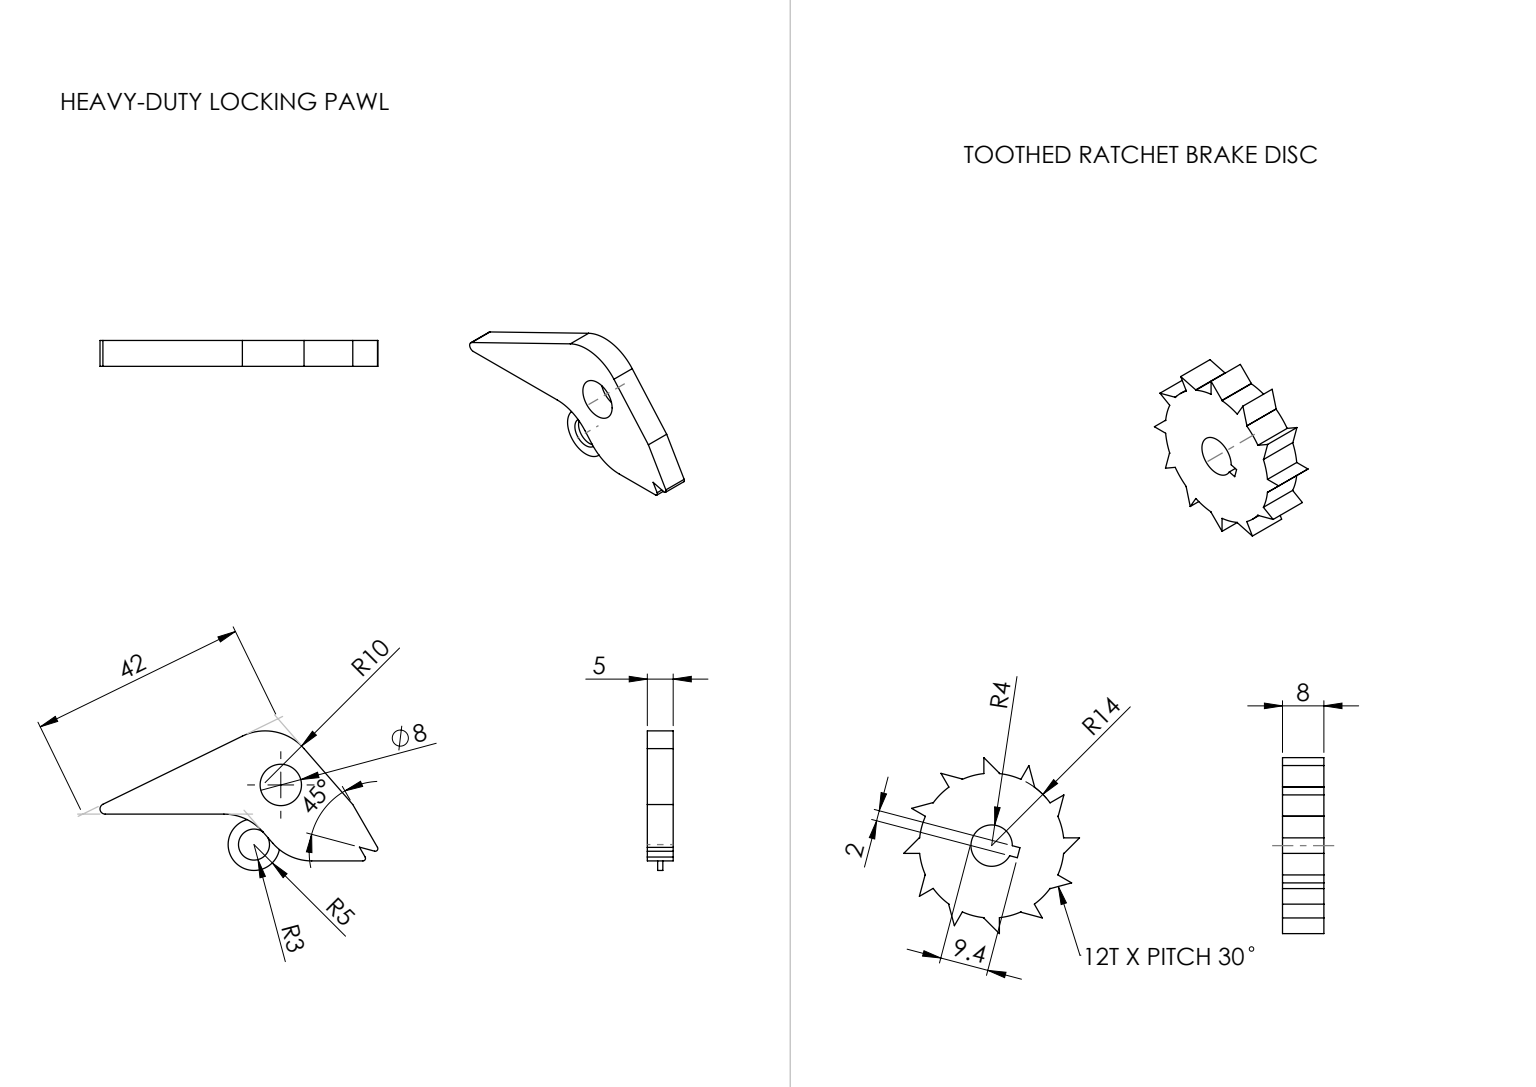
ISO-10303-21;
HEADER;
FILE_DESCRIPTION (('STEP AP214'),
    '1' );
FILE_NAME ('Toothed Ratchet Brake Disc.step',
    '2026-09-28T15:49:00',
    ( '' ),
    ( '' ),
    'SwSTEP 2.0',
    'SolidWorks 2026',
    '' );
FILE_SCHEMA (( 'AUTOMOTIVE_DESIGN' ));
ENDSEC;

DATA;
#67=DIRECTION ( 'NONE',  ( 1.226634733346697831E-16, 0.9659258262890664248, 0.2588190451025275673 ) ) ;
#91=SURFACE_STYLE_FILL_AREA ( #262 ) ;
#100=SURFACE_STYLE_FILL_AREA ( #24773 ) ;
#106=AXIS2_PLACEMENT_3D ( 'NONE', #28368, #3711, #14664 ) ;
#138=VECTOR ( 'NONE', #11051, 999.9999999999998863 ) ;
#168=DIRECTION ( 'NONE',  ( 0.000000000000000000, -2.423959199780483078E-15, 1.000000000000000000 ) ) ;
#214=CARTESIAN_POINT ( 'NONE',  ( -34.49999999999998579, -13.17619866229204284, 90.66066734786082293 ) ) ;
#223=VERTEX_POINT ( 'NONE', #1907 ) ;
#230=EDGE_CURVE ( 'NONE', #16800, #15848, #17909, .T. ) ;
#248=LINE ( 'NONE', #32677, #17648 ) ;
#262=FILL_AREA_STYLE ('',( #8710 ) ) ;
#273=CARTESIAN_POINT ( 'NONE',  ( -21.15833593587365513, -18.77980021920990694, 100.4724318643354053 ) ) ;
#283=CARTESIAN_POINT ( 'NONE',  ( -42.49999999999999289, -34.23950567274748380, 96.30456345124107997 ) ) ;
#289=VECTOR ( 'NONE', #25912, 1000.000000000000000 ) ;
#294=CARTESIAN_POINT ( 'NONE',  ( -42.49999999999999289, -25.98076211353322051, 84.99999999999992895 ) ) ;
#298=CARTESIAN_POINT ( 'NONE',  ( -34.49999999999998579, -28.81745899286249823, 74.41330312067046293 ) ) ;
#300=ADVANCED_FACE ( 'NONE', ( #12882 ), #23862, .F. ) ;
#305=CARTESIAN_POINT ( 'NONE',  ( -21.15833593587365513, -33.18172400785640264, 69.52756813566438154 ) ) ;
#336=ORIENTED_EDGE ( 'NONE', *, *, #17121, .F. ) ;
#370=AXIS2_PLACEMENT_3D ( 'NONE', #13032, #24546, #7606 ) ;
#374=DIRECTION ( 'NONE',  ( -1.226634733346697831E-16, -0.2588190451025116356, -0.9659258262890706437 ) ) ;
#376=EDGE_LOOP ( 'NONE', ( #21433, #15135, #23914, #10868 ) ) ;
#381=DIRECTION ( 'NONE',  ( 1.000000000000000000, 0.000000000000000000, 0.000000000000000000 ) ) ;
#391=ORIENTED_EDGE ( 'NONE', *, *, #34173, .T. ) ;
#484=CARTESIAN_POINT ( 'NONE',  ( -34.49999999999998579, -34.23950567274747669, 96.30456345124106576 ) ) ;
#490=ORIENTED_EDGE ( 'NONE', *, *, #31210, .T. ) ;
#532=VERTEX_POINT ( 'NONE', #20194 ) ;
#590=VECTOR ( 'NONE', #2265, 1000.000000000000000 ) ;
#612=SURFACE_SIDE_STYLE ('',( #91 ) ) ;
#625=DIRECTION ( 'NONE',  ( 0.000000000000000000, 1.000000000000000000, 0.000000000000000000 ) ) ;
#642=CARTESIAN_POINT ( 'NONE',  ( -21.15833593587365513, -14.60640646055094649, 76.70096189432339884 ) ) ;
#659=CARTESIAN_POINT ( 'NONE',  ( -34.49999999999998579, -25.98076211353320986, 84.99999999999994316 ) ) ;
#697=VECTOR ( 'NONE', #11975, 1000.000000000000114 ) ;
#709=VECTOR ( 'NONE', #30336, 1000.000000000000000 ) ;
#713=ORIENTED_EDGE ( 'NONE', *, *, #23446, .F. ) ;
#720=CARTESIAN_POINT ( 'NONE',  ( -42.49999999999999289, -12.06135120645816983, 86.49999999999994316 ) ) ;
#743=EDGE_CURVE ( 'NONE', #35591, #7199, #12479, .T. ) ;
#745=EDGE_CURVE ( 'NONE', #21122, #17030, #7068, .T. ) ;
#746=DIRECTION ( 'NONE',  ( 0.000000000000000000, -0.4999999999999958367, -0.8660254037844410391 ) ) ;
#747=VECTOR ( 'NONE', #16758, 1000.000000000000000 ) ;
#750=EDGE_LOOP ( 'NONE', ( #4388, #25058, #30347, #34872, #28090, #6286 ) ) ;
#767=CARTESIAN_POINT ( 'NONE',  ( -21.15833593587365513, -26.68172400785662290, 89.21410161513769310 ) ) ;
#789=PRESENTATION_STYLE_ASSIGNMENT (( #11768 ) ) ;
#793=VERTEX_POINT ( 'NONE', #28863 ) ;
#820=ORIENTED_EDGE ( 'NONE', *, *, #33243, .T. ) ;
#830=ORIENTED_EDGE ( 'NONE', *, *, #13493, .F. ) ;
#861=CARTESIAN_POINT ( 'NONE',  ( -34.49999999999998579, -25.98076211353322051, 84.99999999999992895 ) ) ;
#872=PRODUCT_DEFINITION_SHAPE ( 'NONE', 'NONE',  #912 ) ;
#874=AXIS2_PLACEMENT_3D ( 'NONE', #19196, #30544, #22421 ) ;
#882=CARTESIAN_POINT ( 'NONE',  ( -34.49999999999998579, -31.64142946139415713, 97.80456345124107997 ) ) ;
#884=ORIENTED_EDGE ( 'NONE', *, *, #5572, .F. ) ;
#912=PRODUCT_DEFINITION ( 'UNKNOWN', '', #34489, #31011 ) ;
#916=LINE ( 'NONE', #17108, #747 ) ;
#930=VECTOR ( 'NONE', #2407, 1000.000000000000114 ) ;
#952=DIRECTION ( 'NONE',  ( 0.000000000000000000, 0.8660254037844444808, -0.4999999999999898415 ) ) ;
#957=UNCERTAINTY_MEASURE_WITH_UNIT (LENGTH_MEASURE( 1.000000000000000082E-05 ), #30348, 'distance_accuracy_value', 'NONE');
#969=DIRECTION ( 'NONE',  ( -1.734723475976807094E-16, 0.8660254037844444808, -0.4999999999999898415 ) ) ;
#1011=CARTESIAN_POINT ( 'NONE',  ( -42.49999999999999289, -28.69486372867094559, 81.70096189432321410 ) ) ;
#1039=ORIENTED_EDGE ( 'NONE', *, *, #33488, .T. ) ;
#1041=CARTESIAN_POINT ( 'NONE',  ( -34.49999999999998579, -25.98076211353322051, 84.99999999999992895 ) ) ;
#1058=DIRECTION ( 'NONE',  ( 0.000000000000000000, -1.000000000000000000, 1.067522139062650474E-15 ) ) ;
#1064=EDGE_CURVE ( 'NONE', #1802, #27521, #4812, .T. ) ;
#1077=CARTESIAN_POINT ( 'NONE',  ( -34.49999999999998579, -25.98076211353322051, 84.99999999999992895 ) ) ;
#1084=FACE_OUTER_BOUND ( 'NONE', #26395, .T. ) ;
#1107=ORIENTED_EDGE ( 'NONE', *, *, #7172, .T. ) ;
#1108=LINE ( 'NONE', #12077, #15873 ) ;
#1118=ORIENTED_EDGE ( 'NONE', *, *, #2748, .F. ) ;
#1133=EDGE_CURVE ( 'NONE', #14117, #4018, #916, .T. ) ;
#1135=DIRECTION ( 'NONE',  ( -1.000000000000000000, -1.734723475976807094E-16, -0.000000000000000000 ) ) ;
#1160=ORIENTED_EDGE ( 'NONE', *, *, #5332, .F. ) ;
#1190=DIRECTION ( 'NONE',  ( -1.000000000000000000, -1.734723475976807094E-16, -0.000000000000000000 ) ) ;
#1231=VECTOR ( 'NONE', #22493, 1000.000000000000000 ) ;
#1252=ORIENTED_EDGE ( 'NONE', *, *, #745, .F. ) ;
#1254=EDGE_CURVE ( 'NONE', #9156, #35591, #5972, .T. ) ;
#1256=VERTEX_POINT ( 'NONE', #17999 ) ;
#1281=ORIENTED_EDGE ( 'NONE', *, *, #9466, .T. ) ;
#1292=CARTESIAN_POINT ( 'NONE',  ( -42.49999999999999289, -27.48076211353326670, 88.99999999999994316 ) ) ;
#1302=DIRECTION ( 'NONE',  ( -1.000000000000000000, 8.673617379884106963E-17, -1.502314598737155580E-16 ) ) ;
#1323=AXIS2_PLACEMENT_3D ( 'NONE', #31219, #31395, #28341 ) ;
#1325=CARTESIAN_POINT ( 'NONE',  ( -34.49999999999998579, -25.98076211353322051, 84.99999999999992895 ) ) ;
#1350=LINE ( 'NONE', #28720, #24089 ) ;
#1363=CARTESIAN_POINT ( 'NONE',  ( -42.49999999999999289, -28.31857036507959791, 80.03062855292519373 ) ) ;
#1377=ORIENTED_EDGE ( 'NONE', *, *, #12991, .T. ) ;
#1445=LINE ( 'NONE', #31682, #19350 ) ;
#1448=VECTOR ( 'NONE', #31600, 1000.000000000000000 ) ;
#1470=CARTESIAN_POINT ( 'NONE',  ( -42.49999999999999289, -39.98076211353324538, 86.49999999999991473 ) ) ;
#1481=VECTOR ( 'NONE', #20731, 1000.000000000000114 ) ;
#1493=PLANE ( 'NONE',  #24055 ) ;
#1540=PLANE ( 'NONE',  #18233 ) ;
#1549=LINE ( 'NONE', #34863, #34826 ) ;
#1578=CARTESIAN_POINT ( 'NONE',  ( -34.49999999999998579, -25.98076211353322051, 84.99999999999992895 ) ) ;
#1582=EDGE_CURVE ( 'NONE', #13818, #6950, #20310, .T. ) ;
#1596=ORIENTED_EDGE ( 'NONE', *, *, #33710, .T. ) ;
#1623=ORIENTED_EDGE ( 'NONE', *, *, #17089, .F. ) ;
#1665=EDGE_CURVE ( 'NONE', #29583, #1876, #28085, .T. ) ;
#1668=EDGE_LOOP ( 'NONE', ( #2169, #17743, #21622, #22182 ) ) ;
#1721=DIRECTION ( 'NONE',  ( -1.000000000000000000, -1.734723475976807094E-16, -0.000000000000000000 ) ) ;
#1722=ORIENTED_EDGE ( 'NONE', *, *, #30631, .F. ) ;
#1723=CARTESIAN_POINT ( 'NONE',  ( -34.49999999999998579, -29.98076211353321341, 84.99999999999994316 ) ) ;
#1745=EDGE_CURVE ( 'NONE', #7407, #24192, #5764, .T. ) ;
#1747=CIRCLE ( 'NONE', #6335, 14.00000000000000000 ) ;
#1771=ORIENTED_EDGE ( 'NONE', *, *, #20086, .T. ) ;
#1772=VECTOR ( 'NONE', #28510, 1000.000000000000000 ) ;
#1790=SHAPE_REPRESENTATION ( 'Toothed Ratchet Brake Disc', ( #21307 ), #24207 ) ;
#1796=EDGE_LOOP ( 'NONE', ( #2648, #490, #8320, #32587 ) ) ;
#1798=LINE ( 'NONE', #15450, #30635 ) ;
#1802=VERTEX_POINT ( 'NONE', #20830 ) ;
#1849=DIRECTION ( 'NONE',  ( -1.734723475976807094E-16, -1.000000000000000000, 1.067522139062650474E-15 ) ) ;
#1861=LINE ( 'NONE', #9769, #1481 ) ;
#1876=VERTEX_POINT ( 'NONE', #34375 ) ;
#1897=CARTESIAN_POINT ( 'NONE',  ( -21.15833593587365513, -17.68172400785659448, 96.37435565298210349 ) ) ;
#1907=CARTESIAN_POINT ( 'NONE',  ( -34.49999999999998579, -20.27980021920970799, 72.12564434701783966 ) ) ;
#1942=CARTESIAN_POINT ( 'NONE',  ( -34.49999999999998579, -25.98076211353322051, 84.99999999999992895 ) ) ;
#1944=LINE ( 'NONE', #4657, #30693 ) ;
#1993=DIRECTION ( 'NONE',  ( -1.734723475976806848E-16, -0.5000000000000032196, 0.8660254037844368202 ) ) ;
#2045=ADVANCED_FACE ( 'NONE', ( #10242 ), #21015, .F. ) ;
#2055=CARTESIAN_POINT ( 'NONE',  ( -21.15833593587365513, -41.45319397786874305, 92.20096189432315725 ) ) ;
#2065=AXIS2_PLACEMENT_3D ( 'NONE', #10185, #21155, #35049 ) ;
#2089=LINE ( 'NONE', #5145, #15629 ) ;
#2128=VECTOR ( 'NONE', #14487, 1000.000000000000114 ) ;
#2135=DIRECTION ( 'NONE',  ( 0.000000000000000000, 1.000000000000000000, 0.000000000000000000 ) ) ;
#2143=DIRECTION ( 'NONE',  ( -1.000000000000000000, 0.000000000000000000, 0.000000000000000000 ) ) ;
#2158=VERTEX_POINT ( 'NONE', #5888 ) ;
#2167=CIRCLE ( 'NONE', #11345, 4.000000000000003553 ) ;
#2169=ORIENTED_EDGE ( 'NONE', *, *, #33690, .T. ) ;
#2219=EDGE_CURVE ( 'NONE', #1802, #4018, #27520, .T. ) ;
#2233=EDGE_LOOP ( 'NONE', ( #14028, #3994, #27129, #18101 ) ) ;
#2265=DIRECTION ( 'NONE',  ( 0.000000000000000000, 0.8660254037844444808, -0.4999999999999898415 ) ) ;
#2267=EDGE_CURVE ( 'NONE', #21074, #13818, #12004, .T. ) ;
#2275=LINE ( 'NONE', #13243, #709 ) ;
#2302=EDGE_CURVE ( 'NONE', #19176, #17996, #9826, .T. ) ;
#2303=FACE_OUTER_BOUND ( 'NONE', #6582, .T. ) ;
#2316=DIRECTION ( 'NONE',  ( -1.000000000000000000, -8.673617379884000959E-17, -1.502314598737161250E-16 ) ) ;
#2346=AXIS2_PLACEMENT_3D ( 'NONE', #11575, #33536, #11404 ) ;
#2383=( GEOMETRIC_REPRESENTATION_CONTEXT ( 3 ) GLOBAL_UNCERTAINTY_ASSIGNED_CONTEXT ( ( #20016 ) ) GLOBAL_UNIT_ASSIGNED_CONTEXT ( ( #33391, #27658, #14121 ) ) REPRESENTATION_CONTEXT ( 'NONE', 'WORKASPACE' ) );
#2407=DIRECTION ( 'NONE',  ( 1.226634733346697831E-16, -0.9659258262890715319, 0.2588190451025083605 ) ) ;
#2456=VERTEX_POINT ( 'NONE', #10009 ) ;
#2462=EDGE_CURVE ( 'NONE', #20834, #17030, #15565, .T. ) ;
#2484=CARTESIAN_POINT ( 'NONE',  ( -21.15833593587365513, -27.48076211353304998, 70.99999999999988631 ) ) ;
#2498=VERTEX_POINT ( 'NONE', #32328 ) ;
#2517=DIRECTION ( 'NONE',  ( -1.000000000000000000, 0.000000000000000000, 0.000000000000000000 ) ) ;
#2520=EDGE_CURVE ( 'NONE', #32530, #7199, #35056, .T. ) ;
#2523=EDGE_CURVE ( 'NONE', #4350, #6950, #13086, .T. ) ;
#2530=CARTESIAN_POINT ( 'NONE',  ( -42.49999999999999289, -29.98076211353323828, 83.49999999999990052 ) ) ;
#2555=AXIS2_PLACEMENT_3D ( 'NONE', #6224, #11791, #31419 ) ;
#2578=VERTEX_POINT ( 'NONE', #3343 ) ;
#2602=CIRCLE ( 'NONE', #11188, 14.00000000000000000 ) ;
#2614=DIRECTION ( 'NONE',  ( -0.000000000000000000, 0.2538061376417689585, 0.9672551082808338307 ) ) ;
#2641=( NAMED_UNIT ( * ) SI_UNIT ( $, .STERADIAN. ) SOLID_ANGLE_UNIT ( ) );
#2648=ORIENTED_EDGE ( 'NONE', *, *, #32954, .F. ) ;
#2650=VECTOR ( 'NONE', #31959, 1000.000000000000000 ) ;
#2655=CIRCLE ( 'NONE', #7232, 4.000000000000003553 ) ;
#2657=CARTESIAN_POINT ( 'NONE',  ( -34.49999999999998579, -36.56745899286261192, 82.16330312067040609 ) ) ;
#2662=DIRECTION ( 'NONE',  ( -1.000000000000000000, -0.000000000000000000, 0.000000000000000000 ) ) ;
#2673=LINE ( 'NONE', #27156, #7841 ) ;
#2700=PLANE ( 'NONE',  #25279 ) ;
#2701=VECTOR ( 'NONE', #3450, 1000.000000000000000 ) ;
#2706=CARTESIAN_POINT ( 'NONE',  ( -34.49999999999998579, -24.48076211353326315, 88.99999999999994316 ) ) ;
#2720=ORIENTED_EDGE ( 'NONE', *, *, #4952, .T. ) ;
#2722=VECTOR ( 'NONE', #8673, 1000.000000000000000 ) ;
#2748=EDGE_CURVE ( 'NONE', #9169, #3468, #3872, .T. ) ;
#2752=EDGE_CURVE ( 'NONE', #17749, #32986, #9426, .T. ) ;
#2788=ORIENTED_EDGE ( 'NONE', *, *, #35495, .T. ) ;
#2813=CARTESIAN_POINT ( 'NONE',  ( -34.49999999999998579, -27.48076211353304643, 71.08058909292485339 ) ) ;
#2832=ADVANCED_FACE ( 'NONE', ( #14460 ), #6373, .T. ) ;
#2851=CARTESIAN_POINT ( 'NONE',  ( -42.49999999999999289, -10.50833024919764469, 77.79903810567677169 ) ) ;
#2857=LINE ( 'NONE', #16320, #15912 ) ;
#2858=DIRECTION ( 'NONE',  ( -0.000000000000000000, -0.2538061376417690140, -0.9672551082808337197 ) ) ;
#2900=ADVANCED_FACE ( 'NONE', ( #31578 ), #17880, .F. ) ;
#2956=ORIENTED_EDGE ( 'NONE', *, *, #21274, .F. ) ;
#2957=ORIENTED_EDGE ( 'NONE', *, *, #8447, .F. ) ;
#2977=DIRECTION ( 'NONE',  ( -1.000000000000000000, -1.817026393327835042E-30, 1.734723475976807094E-16 ) ) ;
#2980=ORIENTED_EDGE ( 'NONE', *, *, #9162, .T. ) ;
#3003=VECTOR ( 'NONE', #14853, 1000.000000000000114 ) ;
#3019=PLANE ( 'NONE',  #23978 ) ;
#3062=ORIENTED_EDGE ( 'NONE', *, *, #8553, .T. ) ;
#3066=LINE ( 'NONE', #10984, #34199 ) ;
#3070=LINE ( 'NONE', #25557, #11972 ) ;
#3079=ORIENTED_EDGE ( 'NONE', *, *, #5513, .T. ) ;
#3093=CARTESIAN_POINT ( 'NONE',  ( -34.49999999999998579, -37.28532556477434667, 76.74125644078563369 ) ) ;
#3099=AXIS2_PLACEMENT_3D ( 'NONE', #15061, #18124, #2135 ) ;
#3101=LINE ( 'NONE', #25050, #12956 ) ;
#3144=DIRECTION ( 'NONE',  ( 0.000000000000000000, 1.000000000000000000, 0.000000000000000000 ) ) ;
#3153=PLANE ( 'NONE',  #7233 ) ;
#3182=VECTOR ( 'NONE', #30896, 1000.000000000000000 ) ;
#3187=CARTESIAN_POINT ( 'NONE',  ( -34.49999999999998579, -25.98076211353322051, 84.99999999999992895 ) ) ;
#3198=VECTOR ( 'NONE', #1993, 999.9999999999998863 ) ;
#3300=VECTOR ( 'NONE', #8931, 1000.000000000000000 ) ;
#3305=ORIENTED_EDGE ( 'NONE', *, *, #19236, .T. ) ;
#3325=LINE ( 'NONE', #19501, #6756 ) ;
#3340=VECTOR ( 'NONE', #4704, 1000.000000000000000 ) ;
#3343=CARTESIAN_POINT ( 'NONE',  ( -42.49999999999999289, -17.72201855431888973, 73.69543654875883476 ) ) ;
#3358=ADVANCED_FACE ( 'NONE', ( #33663 ), #8480, .F. ) ;
#3370=FACE_OUTER_BOUND ( 'NONE', #1796, .T. ) ;
#3375=CARTESIAN_POINT ( 'NONE',  ( -42.49999999999999289, -34.27980021920977549, 73.62564434701768334 ) ) ;
#3417=ORIENTED_EDGE ( 'NONE', *, *, #12189, .T. ) ;
#3424=VERTEX_POINT ( 'NONE', #3093 ) ;
#3430=ORIENTED_EDGE ( 'NONE', *, *, #23446, .T. ) ;
#3450=DIRECTION ( 'NONE',  ( -1.734723475976807094E-16, -1.000000000000000000, 1.067522139062650474E-15 ) ) ;
#3468=VERTEX_POINT ( 'NONE', #720 ) ;
#3482=DIRECTION ( 'NONE',  ( -1.226634733346697831E-16, 0.7071067811865466846, 0.7071067811865483499 ) ) ;
#3506=ADVANCED_FACE ( 'NONE', ( #19616 ), #25227, .F. ) ;
#3510=( NAMED_UNIT ( * ) PLANE_ANGLE_UNIT ( ) SI_UNIT ( $, .RADIAN. ) );
#3539=LINE ( 'NONE', #20238, #2128 ) ;
#3553=DIRECTION ( 'NONE',  ( -1.000000000000000000, 0.000000000000000000, 0.000000000000000000 ) ) ;
#3559=DIRECTION ( 'NONE',  ( 1.000000000000000000, 1.734723475976807094E-16, 0.000000000000000000 ) ) ;
#3563=ORIENTED_EDGE ( 'NONE', *, *, #18312, .F. ) ;
#3584=DIRECTION ( 'NONE',  ( 0.000000000000000000, 1.000000000000000000, 0.000000000000000000 ) ) ;
#3594=ORIENTED_EDGE ( 'NONE', *, *, #28049, .F. ) ;
#3597=CARTESIAN_POINT ( 'NONE',  ( -34.49999999999998579, -26.68172400785662290, 89.21410161513767889 ) ) ;
#3600=AXIS2_PLACEMENT_3D ( 'NONE', #10557, #18296, #13274 ) ;
#3629=DIRECTION ( 'NONE',  ( 1.000000000000000000, 0.000000000000000000, 0.000000000000000000 ) ) ;
#3665=FACE_OUTER_BOUND ( 'NONE', #25437, .T. ) ;
#3694=VERTEX_POINT ( 'NONE', #26294 ) ;
#3711=DIRECTION ( 'NONE',  ( -1.000000000000000000, -1.734723475976807094E-16, -0.000000000000000000 ) ) ;
#3734=CARTESIAN_POINT ( 'NONE',  ( -21.15833593587365513, -29.98076211353323828, 83.49999999999990052 ) ) ;
#3742=EDGE_CURVE ( 'NONE', #28748, #5903, #10614, .T. ) ;
#3755=DIRECTION ( 'NONE',  ( -1.000000000000000000, -1.734723475976807094E-16, -0.000000000000000000 ) ) ;
#3784=DIRECTION ( 'NONE',  ( -1.000000000000000000, -1.502314598737170371E-16, 8.673617379883843187E-17 ) ) ;
#3853=CARTESIAN_POINT ( 'NONE',  ( -34.50000000000001421, -24.48076211353301801, 67.99999999999991473 ) ) ;
#3872=LINE ( 'NONE', #20383, #34097 ) ;
#3890=AXIS2_PLACEMENT_3D ( 'NONE', #22393, #7737, #31916 ) ;
#3894=ORIENTED_EDGE ( 'NONE', *, *, #4681, .F. ) ;
#3911=DIRECTION ( 'NONE',  ( 0.000000000000000000, -0.4999999999999989453, -0.8660254037844392627 ) ) ;
#3951=CARTESIAN_POINT ( 'NONE',  ( -42.49999999999999289, -38.78532556477436088, 79.33933265213893549 ) ) ;
#3953=EDGE_CURVE ( 'NONE', #11172, #20834, #21039, .T. ) ;
#3971=ORIENTED_EDGE ( 'NONE', *, *, #13368, .F. ) ;
#3994=ORIENTED_EDGE ( 'NONE', *, *, #2520, .F. ) ;
#4012=VERTEX_POINT ( 'NONE', #13841 ) ;
#4018=VERTEX_POINT ( 'NONE', #21935 ) ;
#4030=ADVANCED_FACE ( 'NONE', ( #32930 ), #14188, .F. ) ;
#4037=CARTESIAN_POINT ( 'NONE',  ( -21.15833593587365513, -21.98076211353320630, 83.49999999999994316 ) ) ;
#4039=DIRECTION ( 'NONE',  ( -1.734723475976806848E-16, -0.8660254037844350439, -0.5000000000000061062 ) ) ;
#4044=CARTESIAN_POINT ( 'NONE',  ( -21.15833593587365513, -27.48076211353330578, 101.9999999999999432 ) ) ;
#4055=DIRECTION ( 'NONE',  ( -1.000000000000000000, 0.000000000000000000, 0.000000000000000000 ) ) ;
#4076=LINE ( 'NONE', #23301, #31790 ) ;
#4080=ORIENTED_EDGE ( 'NONE', *, *, #33432, .T. ) ;
#4086=DIRECTION ( 'NONE',  ( 0.000000000000000000, 0.9672551082808338307, -0.2538061376417690695 ) ) ;
#4090=CARTESIAN_POINT ( 'NONE',  ( -42.49999999999999289, -27.48076211353330578, 101.9999999999999432 ) ) ;
#4092=AXIS2_PLACEMENT_3D ( 'NONE', #23943, #1135, #23079 ) ;
#4153=ORIENTED_EDGE ( 'NONE', *, *, #25314, .F. ) ;
#4233=AXIS2_PLACEMENT_3D ( 'NONE', #17798, #34393, #9712 ) ;
#4234=ORIENTED_EDGE ( 'NONE', *, *, #24706, .T. ) ;
#4259=DIRECTION ( 'NONE',  ( -1.734723475976807094E-16, 1.000000000000000000, 0.000000000000000000 ) ) ;
#4272=CARTESIAN_POINT ( 'NONE',  ( -34.49999999999998579, -38.78532556477446036, 90.66066734786068082 ) ) ;
#4289=CYLINDRICAL_SURFACE ( 'NONE', #23423, 13.99999999999999822 ) ;
#4290=DIRECTION ( 'NONE',  ( 0.000000000000000000, 1.000000000000000000, 0.000000000000000000 ) ) ;
#4308=ORIENTED_EDGE ( 'NONE', *, *, #9532, .T. ) ;
#4324=ORIENTED_EDGE ( 'NONE', *, *, #33937, .T. ) ;
#4336=CARTESIAN_POINT ( 'NONE',  ( -34.49999999999998579, -21.76666049839546346, 85.70096189432329936 ) ) ;
#4340=LINE ( 'NONE', #21048, #3198 ) ;
#4347=DIRECTION ( 'NONE',  ( 0.000000000000000000, 1.000000000000000000, 0.000000000000000000 ) ) ;
#4348=ORIENTED_EDGE ( 'NONE', *, *, #33937, .F. ) ;
#4350=VERTEX_POINT ( 'NONE', #17008 ) ;
#4360=ORIENTED_EDGE ( 'NONE', *, *, #22271, .F. ) ;
#4372=CARTESIAN_POINT ( 'NONE',  ( -34.49999999999998579, -29.98076211353323473, 86.49999999999990052 ) ) ;
#4388=ORIENTED_EDGE ( 'NONE', *, *, #1064, .T. ) ;
#4409=VECTOR ( 'NONE', #35396, 1000.000000000000000 ) ;
#4420=CARTESIAN_POINT ( 'NONE',  ( -34.49999999999998579, -25.98076211353322051, 84.99999999999992895 ) ) ;
#4446=LINE ( 'NONE', #34143, #26809 ) ;
#4468=CARTESIAN_POINT ( 'NONE',  ( -34.49999999999998579, -23.14406523420388950, 95.58669687932936654 ) ) ;
#4493=ADVANCED_FACE ( 'NONE', ( #22587 ), #25673, .F. ) ;
#4496=CIRCLE ( 'NONE', #3890, 14.00000000000000000 ) ;
#4504=ORIENTED_EDGE ( 'NONE', *, *, #33430, .T. ) ;
#4560=EDGE_LOOP ( 'NONE', ( #10454, #30109, #25468, #18298 ) ) ;
#4567=CARTESIAN_POINT ( 'NONE',  ( -34.49999999999998579, -39.98076211353324538, 86.49999999999991473 ) ) ;
#4568=EDGE_CURVE ( 'NONE', #18652, #34234, #31770, .T. ) ;
#4573=DIRECTION ( 'NONE',  ( 1.000000000000000000, 1.734723475976807094E-16, 0.000000000000000000 ) ) ;
#4604=DIRECTION ( 'NONE',  ( 1.000000000000000000, 1.734723475976807094E-16, 0.000000000000000000 ) ) ;
#4631=CARTESIAN_POINT ( 'NONE',  ( -21.15833593587365513, -38.85511776651532756, 79.29903810567645905 ) ) ;
#4657=CARTESIAN_POINT ( 'NONE',  ( -42.49999999999999289, -30.19486372867095980, 84.29903810567654432 ) ) ;
#4665=LINE ( 'NONE', #7681, #18087 ) ;
#4679=ORIENTED_EDGE ( 'NONE', *, *, #33002, .F. ) ;
#4680=ORIENTED_EDGE ( 'NONE', *, *, #24046, .T. ) ;
#4681=EDGE_CURVE ( 'NONE', #9312, #20546, #15186, .T. ) ;
#4704=DIRECTION ( 'NONE',  ( -1.734723475976807094E-16, 0.8660254037844385966, 0.5000000000000001110 ) ) ;
#4723=EDGE_CURVE ( 'NONE', #6235, #33126, #5973, .T. ) ;
#4726=DIRECTION ( 'NONE',  ( 0.000000000000000000, 0.5000000000000062172, -0.8660254037844351549 ) ) ;
#4733=ORIENTED_EDGE ( 'NONE', *, *, #2523, .F. ) ;
#4759=ADVANCED_FACE ( 'NONE', ( #35564 ), #16437, .T. ) ;
#4774=DIRECTION ( 'NONE',  ( 0.000000000000000000, 0.8660254037844385966, 0.5000000000000001110 ) ) ;
#4784=DIRECTION ( 'NONE',  ( -1.000000000000000000, -8.673617379884210501E-17, 1.502314598737149170E-16 ) ) ;
#4812=CIRCLE ( 'NONE', #19718, 4.000000000000003553 ) ;
#4837=CARTESIAN_POINT ( 'NONE',  ( -34.49999999999998579, -22.68172400785649501, 82.28589838486220742 ) ) ;
#4847=ORIENTED_EDGE ( 'NONE', *, *, #34173, .F. ) ;
#4860=DIRECTION ( 'NONE',  ( 1.000000000000000000, 1.734723475976807094E-16, 0.000000000000000000 ) ) ;
#4862=DIRECTION ( 'NONE',  ( 0.000000000000000000, 1.067522139062650474E-15, 1.000000000000000000 ) ) ;
#4902=EDGE_LOOP ( 'NONE', ( #20074, #26565, #28777, #32466 ) ) ;
#4938=ORIENTED_EDGE ( 'NONE', *, *, #1254, .T. ) ;
#4952=EDGE_CURVE ( 'NONE', #9169, #19399, #18177, .T. ) ;
#4959=LINE ( 'NONE', #33028, #11930 ) ;
#5090=EDGE_CURVE ( 'NONE', #31100, #34028, #10805, .T. ) ;
#5126=AXIS2_PLACEMENT_3D ( 'NONE', #6386, #28352, #625 ) ;
#5145=CARTESIAN_POINT ( 'NONE',  ( -21.15833593587365513, -42.98076211353323828, 83.49999999999991473 ) ) ;
#5161=CARTESIAN_POINT ( 'NONE',  ( -34.49999999999998579, -18.23076211353324183, 92.74999999999997158 ) ) ;
#5200=ORIENTED_EDGE ( 'NONE', *, *, #7172, .F. ) ;
#5220=AXIS2_PLACEMENT_3D ( 'NONE', #767, #6000, #14267 ) ;
#5231=DIRECTION ( 'NONE',  ( 0.000000000000000000, -0.5000000000000092149, 0.8660254037844333785 ) ) ;
#5243=LINE ( 'NONE', #27379, #33207 ) ;
#5332=EDGE_CURVE ( 'NONE', #28748, #25299, #8325, .T. ) ;
#5336=ADVANCED_FACE ( 'NONE', ( #19235 ), #10978, .T. ) ;
#5339=EDGE_LOOP ( 'NONE', ( #13689, #7556, #30424, #9224 ) ) ;
#5389=DIRECTION ( 'NONE',  ( 0.000000000000000000, -0.7071067811865483499, 0.7071067811865466846 ) ) ;
#5423=AXIS2_PLACEMENT_3D ( 'NONE', #9008, #5664, #11062 ) ;
#5459=PLANE ( 'NONE',  #17039 ) ;
#5490=VERTEX_POINT ( 'NONE', #20642 ) ;
#5493=CLOSED_SHELL ( 'NONE', ( #26968, #27749, #28907, #22483, #29677, #13524, #20199, #5336, #7924, #12190, #15124, #8795, #20485, #20576, #27272, #28640, #13379, #17490, #9704, #32827, #29515, #23382, #300, #3358, #28616, #12758, #20945, #24432, #29155, #3506, #20278, #25731, #27800, #4493, #29320, #2045, #9764, #15995, #27342, #34969, #5725, #9052, #20289, #2832, #2900, #31902, #29927, #23062, #34794, #27356, #13730, #4030, #32793, #4759, #7265, #13638 ) ) ;
#5513=EDGE_CURVE ( 'NONE', #31100, #11172, #2602, .T. ) ;
#5531=PLANE ( 'NONE',  #29720 ) ;
#5533=FACE_OUTER_BOUND ( 'NONE', #29475, .T. ) ;
#5572=EDGE_CURVE ( 'NONE', #9519, #12635, #4665, .T. ) ;
#5600=ORIENTED_EDGE ( 'NONE', *, *, #27556, .T. ) ;
#5606=ORIENTED_EDGE ( 'NONE', *, *, #10861, .F. ) ;
#5610=VECTOR ( 'NONE', #19327, 1000.000000000000000 ) ;
#5664=DIRECTION ( 'NONE',  ( 1.000000000000000000, 1.734723475976807094E-16, 0.000000000000000000 ) ) ;
#5673=CARTESIAN_POINT ( 'NONE',  ( -34.49999999999998579, -37.28532556477448168, 93.25874355921402525 ) ) ;
#5725=ADVANCED_FACE ( 'NONE', ( #24968 ), #21901, .T. ) ;
#5726=CARTESIAN_POINT ( 'NONE',  ( -34.49999999999998579, -17.68172400785659448, 96.37435565298210349 ) ) ;
#5727=EDGE_CURVE ( 'NONE', #29093, #34324, #27321, .T. ) ;
#5764=LINE ( 'NONE', #22648, #34171 ) ;
#5774=EDGE_CURVE ( 'NONE', #26460, #223, #27846, .T. ) ;
#5799=EDGE_CURVE ( 'NONE', #35019, #17782, #16665, .T. ) ;
#5805=EDGE_CURVE ( 'NONE', #27165, #35019, #33584, .T. ) ;
#5814=ORIENTED_EDGE ( 'NONE', *, *, #11013, .T. ) ;
#5888=CARTESIAN_POINT ( 'NONE',  ( -42.49999999999999289, -14.67619866229204284, 93.25874355921412473 ) ) ;
#5903=VERTEX_POINT ( 'NONE', #17734 ) ;
#5921=AXIS2_PLACEMENT_3D ( 'NONE', #6133, #21976, #13882 ) ;
#5972=CIRCLE ( 'NONE', #24952, 14.00000000000000000 ) ;
#5973=CIRCLE ( 'NONE', #5423, 14.00000000000000000 ) ;
#6000=DIRECTION ( 'NONE',  ( 0.000000000000000000, -0.8660254037844368202, -0.5000000000000031086 ) ) ;
#6023=VECTOR ( 'NONE', #31614, 1000.000000000000000 ) ;
#6035=EDGE_CURVE ( 'NONE', #20546, #26137, #26573, .T. ) ;
#6049=CYLINDRICAL_SURFACE ( 'NONE', #106, 4.000000000000003553 ) ;
#6089=DIRECTION ( 'NONE',  ( -1.734723475976807094E-16, -2.423959199780483078E-15, 1.000000000000000000 ) ) ;
#6092=LINE ( 'NONE', #12747, #20705 ) ;
#6129=AXIS2_PLACEMENT_3D ( 'NONE', #1325, #26357, #7077 ) ;
#6133=CARTESIAN_POINT ( 'NONE',  ( -21.15833593587365513, -33.18172400785640264, 69.52756813566438154 ) ) ;
#6172=VERTEX_POINT ( 'NONE', #29627 ) ;
#6224=CARTESIAN_POINT ( 'NONE',  ( -21.15833593587365513, -30.19486372867095980, 84.29903810567654432 ) ) ;
#6235=VERTEX_POINT ( 'NONE', #27644 ) ;
#6286=ORIENTED_EDGE ( 'NONE', *, *, #2219, .F. ) ;
#6308=VECTOR ( 'NONE', #19220, 1000.000000000000000 ) ;
#6335=AXIS2_PLACEMENT_3D ( 'NONE', #26756, #13076, #9818 ) ;
#6370=ORIENTED_EDGE ( 'NONE', *, *, #16733, .F. ) ;
#6373=PLANE ( 'NONE',  #1323 ) ;
#6374=ORIENTED_EDGE ( 'NONE', *, *, #3742, .T. ) ;
#6380=EDGE_CURVE ( 'NONE', #6623, #17782, #28158, .T. ) ;
#6386=CARTESIAN_POINT ( 'NONE',  ( -42.49999999999999289, -25.98076211353322051, 84.99999999999992895 ) ) ;
#6410=DIRECTION ( 'NONE',  ( 0.000000000000000000, -1.000000000000000000, 0.000000000000000000 ) ) ;
#6418=ORIENTED_EDGE ( 'NONE', *, *, #5774, .T. ) ;
#6421=PLANE ( 'NONE',  #28630 ) ;
#6448=ORIENTED_EDGE ( 'NONE', *, *, #25788, .F. ) ;
#6463=CARTESIAN_POINT ( 'NONE',  ( -34.49999999999998579, -15.39406523420380069, 82.16330312067053399 ) ) ;
#6504=AXIS2_PLACEMENT_3D ( 'NONE', #30058, #28068, #19416 ) ;
#6511=ORIENTED_EDGE ( 'NONE', *, *, #28401, .T. ) ;
#6526=DIRECTION ( 'NONE',  ( 1.000000000000000000, 1.734723475976807094E-16, 0.000000000000000000 ) ) ;
#6531=CARTESIAN_POINT ( 'NONE',  ( -42.49999999999999289, -25.98076211353322051, 84.99999999999992895 ) ) ;
#6554=DIRECTION ( 'NONE',  ( 0.000000000000000000, 1.000000000000000000, 0.000000000000000000 ) ) ;
#6569=LINE ( 'NONE', #17546, #6695 ) ;
#6582=EDGE_LOOP ( 'NONE', ( #23195, #14934, #21784, #17958 ) ) ;
#6623=VERTEX_POINT ( 'NONE', #23466 ) ;
#6637=LINE ( 'NONE', #6463, #16528 ) ;
#6670=STYLED_ITEM ( 'NONE', ( #789 ), #34526 ) ;
#6695=VECTOR ( 'NONE', #28552, 1000.000000000000000 ) ;
#6739=LINE ( 'NONE', #29429, #30431 ) ;
#6755=LINE ( 'NONE', #34131, #17037 ) ;
#6756=VECTOR ( 'NONE', #8698, 1000.000000000000000 ) ;
#6771=EDGE_CURVE ( 'NONE', #31595, #26460, #27065, .T. ) ;
#6802=CARTESIAN_POINT ( 'NONE',  ( -21.15833593587365513, -37.35511776651544125, 93.29903810567650169 ) ) ;
#6832=ORIENTED_EDGE ( 'NONE', *, *, #9532, .F. ) ;
#6865=EDGE_LOOP ( 'NONE', ( #29214, #1596, #391, #13334 ) ) ;
#6869=EDGE_CURVE ( 'NONE', #34870, #7845, #35527, .T. ) ;
#6894=AXIS2_PLACEMENT_3D ( 'NONE', #32573, #32753, #5231 ) ;
#6897=CARTESIAN_POINT ( 'NONE',  ( -34.49999999999998579, -29.98076211353321341, 84.99999999999994316 ) ) ;
#6903=AXIS2_PLACEMENT_3D ( 'NONE', #23940, #5389, #2517 ) ;
#6923=DIRECTION ( 'NONE',  ( 1.000000000000000000, 0.000000000000000000, 0.000000000000000000 ) ) ;
#6950=VERTEX_POINT ( 'NONE', #28117 ) ;
#6978=DIRECTION ( 'NONE',  ( 0.000000000000000000, 1.000000000000000000, 0.000000000000000000 ) ) ;
#6984=LINE ( 'NONE', #4837, #16954 ) ;
#6989=ORIENTED_EDGE ( 'NONE', *, *, #34831, .F. ) ;
#7000=ORIENTED_EDGE ( 'NONE', *, *, #20746, .T. ) ;
#7003=LINE ( 'NONE', #14746, #27589 ) ;
#7018=CARTESIAN_POINT ( 'NONE',  ( -34.49999999999998579, -28.81745899286270074, 95.58669687932930970 ) ) ;
#7026=CARTESIAN_POINT ( 'NONE',  ( -34.49999999999998579, -25.98076211353322051, 84.99999999999992895 ) ) ;
#7052=LINE ( 'NONE', #9586, #9726 ) ;
#7055=EDGE_CURVE ( 'NONE', #3424, #7407, #1108, .T. ) ;
#7068=LINE ( 'NONE', #9774, #17415 ) ;
#7077=DIRECTION ( 'NONE',  ( 0.000000000000000000, 1.000000000000000000, 0.000000000000000000 ) ) ;
#7082=ORIENTED_EDGE ( 'NONE', *, *, #32457, .T. ) ;
#7135=EDGE_CURVE ( 'NONE', #27859, #28824, #2673, .T. ) ;
#7172=EDGE_CURVE ( 'NONE', #11290, #11685, #13465, .T. ) ;
#7199=VERTEX_POINT ( 'NONE', #34419 ) ;
#7232=AXIS2_PLACEMENT_3D ( 'NONE', #20366, #4573, #20905 ) ;
#7233=AXIS2_PLACEMENT_3D ( 'NONE', #33381, #27987, #20376 ) ;
#7243=CARTESIAN_POINT ( 'NONE',  ( -21.15833593587365513, -18.77980021920990694, 100.4724318643354053 ) ) ;
#7265=ADVANCED_FACE ( 'NONE', ( #8399 ), #16672, .F. ) ;
#7274=EDGE_CURVE ( 'NONE', #223, #19677, #33257, .T. ) ;
#7292=LINE ( 'NONE', #10360, #24571 ) ;
#7320=DIRECTION ( 'NONE',  ( -1.000000000000000000, 0.000000000000000000, 0.000000000000000000 ) ) ;
#7325=ORIENTED_EDGE ( 'NONE', *, *, #33112, .F. ) ;
#7346=APPLICATION_CONTEXT ( 'automotive_design' ) ;
#7407=VERTEX_POINT ( 'NONE', #10882 ) ;
#7448=ORIENTED_EDGE ( 'NONE', *, *, #20746, .F. ) ;
#7454=CARTESIAN_POINT ( 'NONE',  ( -34.49999999999998579, -25.98076211353322051, 84.99999999999992895 ) ) ;
#7469=DIRECTION ( 'NONE',  ( 0.000000000000000000, 0.2538061376417690140, 0.9672551082808337197 ) ) ;
#7479=EDGE_CURVE ( 'NONE', #32761, #28824, #35559, .T. ) ;
#7491=VECTOR ( 'NONE', #23799, 1000.000000000000000 ) ;
#7500=CARTESIAN_POINT ( 'NONE',  ( -34.49999999999998579, -13.10640646055107084, 90.70096189432331357 ) ) ;
#7545=CARTESIAN_POINT ( 'NONE',  ( -21.15833593587365513, -21.98076211353320630, 86.49999999999995737 ) ) ;
#7556=ORIENTED_EDGE ( 'NONE', *, *, #1254, .F. ) ;
#7565=ORIENTED_EDGE ( 'NONE', *, *, #12189, .F. ) ;
#7606=DIRECTION ( 'NONE',  ( 0.000000000000000000, -0.4999999999999989453, -0.8660254037844392627 ) ) ;
#7625=LINE ( 'NONE', #27450, #590 ) ;
#7626=DIRECTION ( 'NONE',  ( 0.000000000000000000, -0.4999999999999928946, -0.8660254037844427044 ) ) ;
#7633=EDGE_LOOP ( 'NONE', ( #10864, #1281, #20210, #12900 ) ) ;
#7650=DIRECTION ( 'NONE',  ( 0.000000000000000000, 1.000000000000000000, 0.000000000000000000 ) ) ;
#7660=DIRECTION ( 'NONE',  ( 1.000000000000000000, 0.000000000000000000, 0.000000000000000000 ) ) ;
#7670=EDGE_CURVE ( 'NONE', #2498, #27165, #30840, .T. ) ;
#7678=CARTESIAN_POINT ( 'NONE',  ( -21.15833593587365513, -35.77980021920998155, 98.97243186433534845 ) ) ;
#7681=CARTESIAN_POINT ( 'NONE',  ( -21.15833593587365513, -24.48076211353301801, 67.99999999999991473 ) ) ;
#7698=PLANE ( 'NONE',  #11967 ) ;
#7737=DIRECTION ( 'NONE',  ( 1.000000000000000000, 1.734723475976807094E-16, 0.000000000000000000 ) ) ;
#7841=VECTOR ( 'NONE', #23421, 1000.000000000000227 ) ;
#7845=VERTEX_POINT ( 'NONE', #7500 ) ;
#7856=DIRECTION ( 'NONE',  ( 0.000000000000000000, -0.2588190451025151329, -0.9659258262890697555 ) ) ;
#7860=CARTESIAN_POINT ( 'NONE',  ( -21.15833593587365513, -26.68172400785650922, 80.78589838486213637 ) ) ;
#7917=DIRECTION ( 'NONE',  ( -0.000000000000000000, -0.2538061376417690140, -0.9672551082808337197 ) ) ;
#7924=ADVANCED_FACE ( 'NONE', ( #26067 ), #4289, .T. ) ;
#7941=ORIENTED_EDGE ( 'NONE', *, *, #743, .F. ) ;
#7945=CARTESIAN_POINT ( 'NONE',  ( -21.15833593587365513, -35.77980021920998155, 98.97243186433534845 ) ) ;
#7951=DIRECTION ( 'NONE',  ( 0.000000000000000000, 1.000000000000000000, 9.406921877466749789E-15 ) ) ;
#7955=EDGE_CURVE ( 'NONE', #14767, #532, #24786, .T. ) ;
#7962=VERTEX_POINT ( 'NONE', #283 ) ;
#7983=DIRECTION ( 'NONE',  ( 0.000000000000000000, 9.406921877466749789E-15, -1.000000000000000000 ) ) ;
#8002=DIRECTION ( 'NONE',  ( 0.000000000000000000, -0.8660254037844385966, -0.5000000000000001110 ) ) ;
#8013=CARTESIAN_POINT ( 'NONE',  ( -42.49999999999999289, -25.98076211353322051, 84.99999999999992895 ) ) ;
#8032=CARTESIAN_POINT ( 'NONE',  ( -34.50000000000001421, -16.18172400785637777, 71.02756813566458050 ) ) ;
#8068=DIRECTION ( 'NONE',  ( 0.000000000000000000, -0.9659258262890689783, 0.2588190451025185190 ) ) ;
#8087=CARTESIAN_POINT ( 'NONE',  ( -34.49999999999998579, -24.48076211353304643, 71.08058909292488181 ) ) ;
#8107=ORIENTED_EDGE ( 'NONE', *, *, #25788, .T. ) ;
#8116=LINE ( 'NONE', #7945, #23499 ) ;
#8117=AXIS2_PLACEMENT_3D ( 'NONE', #1942, #26241, #4290 ) ;
#8147=VERTEX_POINT ( 'NONE', #19618 ) ;
#8245=CARTESIAN_POINT ( 'NONE',  ( -34.49999999999998579, -37.28532556477447457, 93.25874355921401104 ) ) ;
#8276=DIRECTION ( 'NONE',  ( 0.000000000000000000, -0.2588190451025342842, 0.9659258262890646485 ) ) ;
#8277=AXIS2_PLACEMENT_3D ( 'NONE', #25412, #2614, #3629 ) ;
#8320=ORIENTED_EDGE ( 'NONE', *, *, #17121, .T. ) ;
#8325=CIRCLE ( 'NONE', #10054, 14.00000000000000000 ) ;
#8348=EDGE_CURVE ( 'NONE', #9156, #19278, #15104, .T. ) ;
#8365=SURFACE_SIDE_STYLE ('',( #100 ) ) ;
#8379=FACE_OUTER_BOUND ( 'NONE', #34810, .T. ) ;
#8392=FACE_OUTER_BOUND ( 'NONE', #34971, .T. ) ;
#8394=ORIENTED_EDGE ( 'NONE', *, *, #8882, .T. ) ;
#8399=FACE_OUTER_BOUND ( 'NONE', #24805, .T. ) ;
#8447=EDGE_CURVE ( 'NONE', #11290, #7845, #18357, .T. ) ;
#8455=DIRECTION ( 'NONE',  ( -1.734723475976806848E-16, -0.5000000000000032196, 0.8660254037844368202 ) ) ;
#8480=PLANE ( 'NONE',  #30618 ) ;
#8553=EDGE_CURVE ( 'NONE', #2578, #27197, #35551, .T. ) ;
#8575=DIRECTION ( 'NONE',  ( -1.226634733346697831E-16, 0.9659258262890715319, -0.2588190451025083605 ) ) ;
#8579=CARTESIAN_POINT ( 'NONE',  ( -34.49999999999998579, -29.27980021920982523, 82.28589838486210795 ) ) ;
#8623=DIRECTION ( 'NONE',  ( -1.000000000000000000, 0.000000000000000000, -0.000000000000000000 ) ) ;
#8635=LINE ( 'NONE', #8807, #1231 ) ;
#8654=CARTESIAN_POINT ( 'NONE',  ( -34.49999999999998579, -27.48076211353314591, 80.99999999999988631 ) ) ;
#8673=DIRECTION ( 'NONE',  ( -1.000000000000000000, 6.056754644426116516E-31, -1.734723475976807094E-16 ) ) ;
#8698=DIRECTION ( 'NONE',  ( -1.000000000000000000, 0.000000000000000000, 0.000000000000000000 ) ) ;
#8710=FILL_AREA_STYLE_COLOUR ( '', #29124 ) ;
#8752=AXIS2_PLACEMENT_3D ( 'NONE', #13622, #16123, #27140 ) ;
#8761=ORIENTED_EDGE ( 'NONE', *, *, #1582, .T. ) ;
#8795=ADVANCED_FACE ( 'NONE', ( #17587 ), #20282, .T. ) ;
#8803=VERTEX_POINT ( 'NONE', #12381 ) ;
#8807=CARTESIAN_POINT ( 'NONE',  ( -42.49999999999999289, -27.48076211353314591, 80.99999999999987210 ) ) ;
#8858=CARTESIAN_POINT ( 'NONE',  ( -34.49999999999998579, -18.23076211353320275, 77.24999999999991473 ) ) ;
#8871=EDGE_CURVE ( 'NONE', #31100, #6235, #21363, .T. ) ;
#8875=DIRECTION ( 'NONE',  ( 0.000000000000000000, 1.000000000000000000, 0.000000000000000000 ) ) ;
#8882=EDGE_CURVE ( 'NONE', #3424, #29247, #31637, .T. ) ;
#8885=CARTESIAN_POINT ( 'NONE',  ( -34.49999999999998579, -25.98076211353320986, 84.99999999999994316 ) ) ;
#8917=DIRECTION ( 'NONE',  ( 0.000000000000000000, -1.000000000000000000, 0.000000000000000000 ) ) ;
#8925=DIRECTION ( 'NONE',  ( -0.000000000000000000, 0.2588190451025275673, -0.9659258262890664248 ) ) ;
#8931=DIRECTION ( 'NONE',  ( -1.000000000000000000, 0.000000000000000000, -0.000000000000000000 ) ) ;
#8962=ORIENTED_EDGE ( 'NONE', *, *, #18274, .T. ) ;
#9008=CARTESIAN_POINT ( 'NONE',  ( -42.49999999999999289, -25.98076211353322051, 84.99999999999992895 ) ) ;
#9034=VECTOR ( 'NONE', #23328, 1000.000000000000000 ) ;
#9039=EDGE_LOOP ( 'NONE', ( #15141, #22315, #25655, #23018 ) ) ;
#9052=ADVANCED_FACE ( 'NONE', ( #29489 ), #18127, .F. ) ;
#9070=CARTESIAN_POINT ( 'NONE',  ( -34.49999999999998579, -33.73076211353313880, 77.24999999999981526 ) ) ;
#9101=VECTOR ( 'NONE', #7320, 1000.000000000000000 ) ;
#9114=CARTESIAN_POINT ( 'NONE',  ( -34.49999999999998579, -25.98076211353322051, 84.99999999999992895 ) ) ;
#9156=VERTEX_POINT ( 'NONE', #10932 ) ;
#9162=EDGE_CURVE ( 'NONE', #1256, #4012, #11274, .T. ) ;
#9165=ORIENTED_EDGE ( 'NONE', *, *, #5090, .T. ) ;
#9169=VERTEX_POINT ( 'NONE', #27317 ) ;
#9224=ORIENTED_EDGE ( 'NONE', *, *, #5332, .T. ) ;
#9262=ORIENTED_EDGE ( 'NONE', *, *, #32174, .T. ) ;
#9290=VECTOR ( 'NONE', #1849, 1000.000000000000000 ) ;
#9294=CYLINDRICAL_SURFACE ( 'NONE', #23287, 13.99999999999999822 ) ;
#9312=VERTEX_POINT ( 'NONE', #16441 ) ;
#9326=EDGE_CURVE ( 'NONE', #23698, #17749, #4959, .T. ) ;
#9420=EDGE_CURVE ( 'NONE', #16181, #793, #29805, .T. ) ;
#9426=LINE ( 'NONE', #23282, #18570 ) ;
#9441=DIRECTION ( 'NONE',  ( 0.000000000000000000, 1.000000000000000000, 0.000000000000000000 ) ) ;
#9455=DIRECTION ( 'NONE',  ( 0.000000000000000000, 0.8660254037844385966, 0.5000000000000001110 ) ) ;
#9462=EDGE_CURVE ( 'NONE', #26147, #12715, #248, .T. ) ;
#9466=EDGE_CURVE ( 'NONE', #26081, #30439, #2167, .T. ) ;
#9513=ORIENTED_EDGE ( 'NONE', *, *, #743, .T. ) ;
#9519=VERTEX_POINT ( 'NONE', #3853 ) ;
#9522=VECTOR ( 'NONE', #19485, 999.9999999999998863 ) ;
#9532=EDGE_CURVE ( 'NONE', #34282, #1802, #3325, .T. ) ;
#9582=AXIS2_PLACEMENT_3D ( 'NONE', #3187, #1190, #8917 ) ;
#9586=CARTESIAN_POINT ( 'NONE',  ( -34.49999999999998579, -34.23950567274748380, 96.30456345124107997 ) ) ;
#9598=DIRECTION ( 'NONE',  ( -1.734723475976807094E-16, -2.423959199780483078E-15, 1.000000000000000000 ) ) ;
#9632=VECTOR ( 'NONE', #27118, 1000.000000000000000 ) ;
#9637=ORIENTED_EDGE ( 'NONE', *, *, #22684, .F. ) ;
#9678=CIRCLE ( 'NONE', #28653, 4.000000000000003553 ) ;
#9703=CYLINDRICAL_SURFACE ( 'NONE', #24037, 13.99999999999999822 ) ;
#9704=ADVANCED_FACE ( 'NONE', ( #23461 ), #14983, .F. ) ;
#9712=DIRECTION ( 'NONE',  ( 0.000000000000000000, -0.8660254037844444808, 0.4999999999999898415 ) ) ;
#9715=VERTEX_POINT ( 'NONE', #20736 ) ;
#9726=VECTOR ( 'NONE', #1302, 1000.000000000000000 ) ;
#9764=ADVANCED_FACE ( 'NONE', ( #34805 ), #1493, .F. ) ;
#9769=CARTESIAN_POINT ( 'NONE',  ( -34.49999999999998579, -25.01350700525237514, 84.74619386235816876 ) ) ;
#9774=CARTESIAN_POINT ( 'NONE',  ( -34.49999999999998579, -27.48076211353326670, 88.99999999999994316 ) ) ;
#9776=ORIENTED_EDGE ( 'NONE', *, *, #14942, .T. ) ;
#9814=DIRECTION ( 'NONE',  ( 0.000000000000000000, 0.9672551082808337197, -0.2538061376417689030 ) ) ;
#9818=DIRECTION ( 'NONE',  ( 0.000000000000000000, 1.000000000000000000, 0.000000000000000000 ) ) ;
#9826=LINE ( 'NONE', #34327, #34194 ) ;
#9834=CARTESIAN_POINT ( 'NONE',  ( -21.15833593587365513, -10.50833024919764469, 77.79903810567677169 ) ) ;
#9842=CARTESIAN_POINT ( 'NONE',  ( -42.49999999999999289, -37.28532556477448168, 93.25874355921402525 ) ) ;
#9843=DIRECTION ( 'NONE',  ( 0.000000000000000000, -1.000000000000000000, 0.000000000000000000 ) ) ;
#9870=ORIENTED_EDGE ( 'NONE', *, *, #2462, .T. ) ;
#9895=ORIENTED_EDGE ( 'NONE', *, *, #11093, .T. ) ;
#9925=CARTESIAN_POINT ( 'NONE',  ( -34.49999999999998579, -33.73076211353324538, 92.74999999999992895 ) ) ;
#9967=ORIENTED_EDGE ( 'NONE', *, *, #14172, .T. ) ;
#9988=ORIENTED_EDGE ( 'NONE', *, *, #13368, .T. ) ;
#10009=CARTESIAN_POINT ( 'NONE',  ( -42.49999999999999289, -31.68172400785665488, 97.87435565298206086 ) ) ;
#10054=AXIS2_PLACEMENT_3D ( 'NONE', #32937, #28244, #3584 ) ;
#10089=AXIS2_PLACEMENT_3D ( 'NONE', #25506, #28560, #3911 ) ;
#10100=ORIENTED_EDGE ( 'NONE', *, *, #13770, .F. ) ;
#10120=( GEOMETRIC_REPRESENTATION_CONTEXT ( 3 ) GLOBAL_UNCERTAINTY_ASSIGNED_CONTEXT ( ( #957 ) ) GLOBAL_UNIT_ASSIGNED_CONTEXT ( ( #30348, #3510, #14458 ) ) REPRESENTATION_CONTEXT ( 'NONE', 'WORKASPACE' ) );
#10185=CARTESIAN_POINT ( 'NONE',  ( -34.49999999999998579, -25.98076211353322051, 84.99999999999992895 ) ) ;
#10192=CARTESIAN_POINT ( 'NONE',  ( -34.49999999999998579, -38.78532556477436088, 79.33933265213893549 ) ) ;
#10214=VERTEX_POINT ( 'NONE', #34719 ) ;
#10230=DIRECTION ( 'NONE',  ( -1.226634733346697831E-16, 0.9659258262890646485, 0.2588190451025342842 ) ) ;
#10242=FACE_OUTER_BOUND ( 'NONE', #4560, .T. ) ;
#10246=AXIS2_PLACEMENT_3D ( 'NONE', #4037, #34455, #34087 ) ;
#10255=VERTEX_POINT ( 'NONE', #26794 ) ;
#10304=CIRCLE ( 'NONE', #13170, 14.00000000000000000 ) ;
#10360=CARTESIAN_POINT ( 'NONE',  ( -42.49999999999999289, -26.68172400785650922, 80.78589838486213637 ) ) ;
#10386=CARTESIAN_POINT ( 'NONE',  ( -34.49999999999998579, -21.76666049839542794, 84.29903810567665801 ) ) ;
#10416=DIRECTION ( 'NONE',  ( 0.000000000000000000, -1.000000000000000000, 0.000000000000000000 ) ) ;
#10425=EDGE_CURVE ( 'NONE', #26694, #5490, #11622, .T. ) ;
#10449=EDGE_LOOP ( 'NONE', ( #27959, #3430, #12857, #13771, #15049, #30958, #23148, #4080, #25336, #3079, #28708, #9870, #1252, #21396, #18668, #3417, #14645, #5600, #27257, #21470, #3971, #7000, #14575, #19709, #33429, #4938, #9513, #4234, #26086, #13877, #32730, #12938, #23941, #12001, #12546, #17746, #15116, #2788, #34508, #27253, #14218, #24494, #10559, #6511, #30430, #12408, #18053, #27441 ) ) ;
#10454=ORIENTED_EDGE ( 'NONE', *, *, #30788, .F. ) ;
#10464=ORIENTED_EDGE ( 'NONE', *, *, #6771, .T. ) ;
#10503=ORIENTED_EDGE ( 'NONE', *, *, #16074, .F. ) ;
#10511=LINE ( 'NONE', #18966, #20034 ) ;
#10557=CARTESIAN_POINT ( 'NONE',  ( -21.15833593587365513, -24.48076211353326315, 88.99999999999994316 ) ) ;
#10559=ORIENTED_EDGE ( 'NONE', *, *, #6380, .T. ) ;
#10592=ORIENTED_EDGE ( 'NONE', *, *, #22499, .F. ) ;
#10614=LINE ( 'NONE', #2530, #32940 ) ;
#10637=EDGE_CURVE ( 'NONE', #3424, #30700, #1747, .T. ) ;
#10640=FACE_OUTER_BOUND ( 'NONE', #30525, .T. ) ;
#10665=PLANE ( 'NONE',  #11782 ) ;
#10677=DIRECTION ( 'NONE',  ( -1.000000000000000000, -0.000000000000000000, 0.000000000000000000 ) ) ;
#10696=CYLINDRICAL_SURFACE ( 'NONE', #19542, 13.99999999999999822 ) ;
#10726=ORIENTED_EDGE ( 'NONE', *, *, #34096, .F. ) ;
#10781=AXIS2_PLACEMENT_3D ( 'NONE', #7678, #7856, #2662 ) ;
#10805=LINE ( 'NONE', #15816, #14614 ) ;
#10806=ORIENTED_EDGE ( 'NONE', *, *, #30517, .T. ) ;
#10861=EDGE_CURVE ( 'NONE', #4012, #9519, #25103, .T. ) ;
#10864=ORIENTED_EDGE ( 'NONE', *, *, #11093, .F. ) ;
#10868=ORIENTED_EDGE ( 'NONE', *, *, #19386, .F. ) ;
#10882=CARTESIAN_POINT ( 'NONE',  ( -34.50000000000001421, -39.95319397786859383, 75.20096189432314304 ) ) ;
#10907=EDGE_LOOP ( 'NONE', ( #17159, #14592, #6989, #27979 ) ) ;
#10932=CARTESIAN_POINT ( 'NONE',  ( -34.49999999999998579, -39.90017302060827831, 83.49999999999991473 ) ) ;
#10946=ORIENTED_EDGE ( 'NONE', *, *, #17089, .T. ) ;
#10978=CYLINDRICAL_SURFACE ( 'NONE', #12340, 13.99999999999999822 ) ;
#10984=CARTESIAN_POINT ( 'NONE',  ( -42.49999999999999289, -24.48076211353326315, 88.99999999999994316 ) ) ;
#10997=VECTOR ( 'NONE', #3784, 1000.000000000000000 ) ;
#11000=ORIENTED_EDGE ( 'NONE', *, *, #20898, .T. ) ;
#11013=EDGE_CURVE ( 'NONE', #6235, #32406, #20026, .T. ) ;
#11021=EDGE_CURVE ( 'NONE', #17030, #26694, #17512, .T. ) ;
#11037=CARTESIAN_POINT ( 'NONE',  ( -34.49999999999998579, -24.48076211353329157, 98.91941090707499029 ) ) ;
#11044=ORIENTED_EDGE ( 'NONE', *, *, #2523, .T. ) ;
#11051=DIRECTION ( 'NONE',  ( 0.000000000000000000, -0.5000000000000032196, 0.8660254037844368202 ) ) ;
#11062=DIRECTION ( 'NONE',  ( 0.000000000000000000, 1.000000000000000000, 0.000000000000000000 ) ) ;
#11068=LINE ( 'NONE', #21679, #15341 ) ;
#11091=CARTESIAN_POINT ( 'NONE',  ( -34.50000000000001421, -42.98076211353323828, 83.49999999999991473 ) ) ;
#11093=EDGE_CURVE ( 'NONE', #26081, #14212, #23468, .T. ) ;
#11119=ORIENTED_EDGE ( 'NONE', *, *, #33112, .T. ) ;
#11124=ORIENTED_EDGE ( 'NONE', *, *, #2462, .F. ) ;
#11172=VERTEX_POINT ( 'NONE', #12670 ) ;
#11173=ORIENTED_EDGE ( 'NONE', *, *, #16267, .T. ) ;
#11188=AXIS2_PLACEMENT_3D ( 'NONE', #861, #15425, #6978 ) ;
#11192=DIRECTION ( 'NONE',  ( 1.000000000000000000, 1.734723475976807094E-16, 0.000000000000000000 ) ) ;
#11210=ORIENTED_EDGE ( 'NONE', *, *, #17748, .F. ) ;
#11224=PLANE ( 'NONE',  #5220 ) ;
#11274=LINE ( 'NONE', #2484, #20523 ) ;
#11279=DIRECTION ( 'NONE',  ( 0.000000000000000000, 0.4999999999999929501, 0.8660254037844428154 ) ) ;
#11282=DIRECTION ( 'NONE',  ( 1.000000000000000000, 1.734723475976807094E-16, 0.000000000000000000 ) ) ;
#11290=VERTEX_POINT ( 'NONE', #214 ) ;
#11293=CARTESIAN_POINT ( 'NONE',  ( -21.15833593587365513, -16.18172400785637777, 71.02756813566458050 ) ) ;
#11334=ORIENTED_EDGE ( 'NONE', *, *, #16733, .T. ) ;
#11345=AXIS2_PLACEMENT_3D ( 'NONE', #18623, #15915, #26932 ) ;
#11359=ORIENTED_EDGE ( 'NONE', *, *, #16074, .T. ) ;
#11364=DIRECTION ( 'NONE',  ( 0.000000000000000000, 0.2588190451025084160, 0.9659258262890716429 ) ) ;
#11391=FACE_OUTER_BOUND ( 'NONE', #1668, .T. ) ;
#11404=DIRECTION ( 'NONE',  ( 0.000000000000000000, 0.4999999999999929501, 0.8660254037844428154 ) ) ;
#11413=VERTEX_POINT ( 'NONE', #22692 ) ;
#11434=PRESENTATION_STYLE_ASSIGNMENT (( #26769 ) ) ;
#11453=DIRECTION ( 'NONE',  ( -1.734723475976806848E-16, -0.8660254037844410391, 0.4999999999999958367 ) ) ;
#11542=LINE ( 'NONE', #8654, #29616 ) ;
#11575=CARTESIAN_POINT ( 'NONE',  ( -21.15833593587365513, -29.27980021920983944, 82.28589838486210795 ) ) ;
#11620=DIRECTION ( 'NONE',  ( 1.000000000000000000, 0.000000000000000000, 0.000000000000000000 ) ) ;
#11622=LINE ( 'NONE', #4090, #23558 ) ;
#11633=DIRECTION ( 'NONE',  ( -1.000000000000000000, 0.000000000000000000, 0.000000000000000000 ) ) ;
#11685=VERTEX_POINT ( 'NONE', #14352 ) ;
#11768=SURFACE_STYLE_USAGE ( .BOTH. , #612 ) ;
#11772=ORIENTED_EDGE ( 'NONE', *, *, #26918, .F. ) ;
#11776=SHAPE_REPRESENTATION_RELATIONSHIP ( 'NONE' , 'NONE' ,  #1790, #17621 ) ;
#11779=DIRECTION ( 'NONE',  ( -1.000000000000000000, 0.000000000000000000, 0.000000000000000000 ) ) ;
#11782=AXIS2_PLACEMENT_3D ( 'NONE', #29228, #7951, #27057 ) ;
#11785=DIRECTION ( 'NONE',  ( 1.000000000000000000, 1.734723475976807094E-16, 0.000000000000000000 ) ) ;
#11791=DIRECTION ( 'NONE',  ( 0.000000000000000000, 0.5000000000000062172, -0.8660254037844351549 ) ) ;
#11819=SHAPE_DEFINITION_REPRESENTATION ( #872, #1790 ) ;
#11851=VECTOR ( 'NONE', #10230, 1000.000000000000000 ) ;
#11869=CARTESIAN_POINT ( 'NONE',  ( -34.49999999999998579, -20.32009476567239048, 97.80456345124113682 ) ) ;
#11872=ORIENTED_EDGE ( 'NONE', *, *, #20292, .F. ) ;
#11887=EDGE_LOOP ( 'NONE', ( #4348, #16409, #14464, #3062 ) ) ;
#11906=EDGE_CURVE ( 'NONE', #4350, #17135, #12461, .T. ) ;
#11917=AXIS2_PLACEMENT_3D ( 'NONE', #8013, #23880, #7650 ) ;
#11930=VECTOR ( 'NONE', #18981, 1000.000000000000000 ) ;
#11931=VECTOR ( 'NONE', #16122, 1000.000000000000227 ) ;
#11962=DIRECTION ( 'NONE',  ( 0.000000000000000000, -0.7071067811865442421, -0.7071067811865509034 ) ) ;
#11967=AXIS2_PLACEMENT_3D ( 'NONE', #18682, #29682, #35274 ) ;
#11972=VECTOR ( 'NONE', #30771, 1000.000000000000114 ) ;
#11975=DIRECTION ( 'NONE',  ( 1.226634733346697831E-16, 0.2588190451025116356, 0.9659258262890706437 ) ) ;
#12001=ORIENTED_EDGE ( 'NONE', *, *, #24318, .T. ) ;
#12004=LINE ( 'NONE', #4272, #6023 ) ;
#12040=CARTESIAN_POINT ( 'NONE',  ( -34.49999999999998579, -26.68172400785649856, 80.78589838486213637 ) ) ;
#12045=FACE_OUTER_BOUND ( 'NONE', #11887, .T. ) ;
#12055=PLANE ( 'NONE',  #12065 ) ;
#12065=AXIS2_PLACEMENT_3D ( 'NONE', #32214, #8068, #35112 ) ;
#12077=CARTESIAN_POINT ( 'NONE',  ( -34.49999999999998579, -28.69486372867093849, 81.70096189432322831 ) ) ;
#12083=ORIENTED_EDGE ( 'NONE', *, *, #24046, .F. ) ;
#12095=DIRECTION ( 'NONE',  ( -1.226634733346697831E-16, -0.7071067811865466846, -0.7071067811865483499 ) ) ;
#12189=EDGE_CURVE ( 'NONE', #1876, #27933, #31276, .T. ) ;
#12190=ADVANCED_FACE ( 'NONE', ( #17395 ), #18115, .T. ) ;
#12216=CARTESIAN_POINT ( 'NONE',  ( -42.49999999999999289, -8.980762113533204527, 86.49999999999994316 ) ) ;
#12285=CARTESIAN_POINT ( 'NONE',  ( -42.49999999999999289, -25.98076211353322051, 84.99999999999992895 ) ) ;
#12301=FACE_OUTER_BOUND ( 'NONE', #14684, .T. ) ;
#12326=DIRECTION ( 'NONE',  ( -1.000000000000000000, 0.000000000000000000, -0.000000000000000000 ) ) ;
#12340=AXIS2_PLACEMENT_3D ( 'NONE', #14017, #30586, #30239 ) ;
#12372=DIRECTION ( 'NONE',  ( -1.000000000000000000, -1.734723475976807094E-16, -0.000000000000000000 ) ) ;
#12377=CARTESIAN_POINT ( 'NONE',  ( -42.49999999999999289, -18.77980021920990694, 100.4724318643354053 ) ) ;
#12381=CARTESIAN_POINT ( 'NONE',  ( -34.50000000000001421, -10.50833024919764469, 77.79903810567677169 ) ) ;
#12408=ORIENTED_EDGE ( 'NONE', *, *, #32954, .T. ) ;
#12427=DIRECTION ( 'NONE',  ( -1.000000000000000000, 8.673617379883896189E-17, 1.502314598737167413E-16 ) ) ;
#12461=LINE ( 'NONE', #4372, #9290 ) ;
#12470=AXIS2_PLACEMENT_3D ( 'NONE', #34130, #20412, #15917 ) ;
#12472=VECTOR ( 'NONE', #2316, 1000.000000000000000 ) ;
#12477=DIRECTION ( 'NONE',  ( 0.000000000000000000, -1.067522139062650474E-15, -1.000000000000000000 ) ) ;
#12479=LINE ( 'NONE', #25989, #32966 ) ;
#12522=FACE_OUTER_BOUND ( 'NONE', #12716, .T. ) ;
#12546=ORIENTED_EDGE ( 'NONE', *, *, #24656, .T. ) ;
#12550=ORIENTED_EDGE ( 'NONE', *, *, #13609, .T. ) ;
#12567=CARTESIAN_POINT ( 'NONE',  ( -34.49999999999998579, -20.32009476567239048, 97.80456345124112261 ) ) ;
#12589=DIRECTION ( 'NONE',  ( -1.226634733346698078E-16, 0.2588190451025185190, 0.9659258262890689783 ) ) ;
#12635=VERTEX_POINT ( 'NONE', #32405 ) ;
#12661=ORIENTED_EDGE ( 'NONE', *, *, #4568, .T. ) ;
#12670=CARTESIAN_POINT ( 'NONE',  ( -34.49999999999998579, -24.48076211353329157, 98.91941090707499029 ) ) ;
#12704=DIRECTION ( 'NONE',  ( 0.000000000000000000, -0.4999999999999928946, -0.8660254037844427044 ) ) ;
#12714=CARTESIAN_POINT ( 'NONE',  ( -42.49999999999999289, -29.98076211353321341, 84.99999999999994316 ) ) ;
#12715=VERTEX_POINT ( 'NONE', #22294 ) ;
#12716=EDGE_LOOP ( 'NONE', ( #17306, #23208, #23005, #24943 ) ) ;
#12725=DIRECTION ( 'NONE',  ( 0.000000000000000000, 0.000000000000000000, 1.000000000000000000 ) ) ;
#12737=CARTESIAN_POINT ( 'NONE',  ( -42.49999999999999289, -17.68172400785659448, 96.37435565298210349 ) ) ;
#12745=VECTOR ( 'NONE', #26058, 1000.000000000000000 ) ;
#12747=CARTESIAN_POINT ( 'NONE',  ( -42.49999999999999289, -21.98076211353320630, 86.49999999999995737 ) ) ;
#12754=FACE_OUTER_BOUND ( 'NONE', #33986, .T. ) ;
#12756=ORIENTED_EDGE ( 'NONE', *, *, #24984, .T. ) ;
#12758=ADVANCED_FACE ( 'NONE', ( #32933 ), #16539, .T. ) ;
#12775=DIRECTION ( 'NONE',  ( -1.000000000000000000, 8.673617379884106963E-17, -1.502314598737155580E-16 ) ) ;
#12792=DIRECTION ( 'NONE',  ( -1.734723475976807094E-16, 1.000000000000000000, -1.067522139062650474E-15 ) ) ;
#12857=ORIENTED_EDGE ( 'NONE', *, *, #8447, .T. ) ;
#12882=FACE_OUTER_BOUND ( 'NONE', #29692, .T. ) ;
#12900=ORIENTED_EDGE ( 'NONE', *, *, #21810, .F. ) ;
#12906=LINE ( 'NONE', #9834, #9101 ) ;
#12929=ORIENTED_EDGE ( 'NONE', *, *, #16723, .T. ) ;
#12938=ORIENTED_EDGE ( 'NONE', *, *, #7955, .T. ) ;
#12946=AXIS2_PLACEMENT_3D ( 'NONE', #34723, #21372, #10416 ) ;
#12956=VECTOR ( 'NONE', #374, 1000.000000000000114 ) ;
#12987=CARTESIAN_POINT ( 'NONE',  ( -21.15833593587365513, -28.69486372867094559, 81.70096189432321410 ) ) ;
#12991=EDGE_CURVE ( 'NONE', #6950, #15285, #14529, .T. ) ;
#13016=CARTESIAN_POINT ( 'NONE',  ( -34.49999999999998579, -13.17619866229195047, 79.33933265213923391 ) ) ;
#13019=DIRECTION ( 'NONE',  ( 0.000000000000000000, 1.000000000000000000, -1.067522139062650474E-15 ) ) ;
#13030=ORIENTED_EDGE ( 'NONE', *, *, #5572, .T. ) ;
#13032=CARTESIAN_POINT ( 'NONE',  ( -21.15833593587365513, -22.68172400785658382, 87.71410161513770731 ) ) ;
#13039=EDGE_CURVE ( 'NONE', #3468, #26771, #6092, .T. ) ;
#13076=DIRECTION ( 'NONE',  ( 1.000000000000000000, 1.734723475976807094E-16, 0.000000000000000000 ) ) ;
#13086=LINE ( 'NONE', #26585, #15646 ) ;
#13170=AXIS2_PLACEMENT_3D ( 'NONE', #31758, #23668, #34654 ) ;
#13184=ORIENTED_EDGE ( 'NONE', *, *, #5799, .T. ) ;
#13210=LINE ( 'NONE', #2055, #33175 ) ;
#13232=DIRECTION ( 'NONE',  ( 0.000000000000000000, -1.000000000000000000, 0.000000000000000000 ) ) ;
#13243=CARTESIAN_POINT ( 'NONE',  ( 75.00000000000001421, -27.93100416606583991, 81.50764321173598148 ) ) ;
#13261=DIRECTION ( 'NONE',  ( -1.226634733346697831E-16, -0.7071067811865507924, 0.7071067811865441310 ) ) ;
#13274=DIRECTION ( 'NONE',  ( 0.000000000000000000, 2.423959199780483078E-15, -1.000000000000000000 ) ) ;
#13313=EDGE_LOOP ( 'NONE', ( #4733, #7448, #34111, #8761 ) ) ;
#13334=ORIENTED_EDGE ( 'NONE', *, *, #13609, .F. ) ;
#13368=EDGE_CURVE ( 'NONE', #21074, #10214, #6755, .T. ) ;
#13379=ADVANCED_FACE ( 'NONE', ( #3370 ), #22776, .T. ) ;
#13411=CARTESIAN_POINT ( 'NONE',  ( -34.49999999999998579, -31.64142946139395107, 72.19543654875866423 ) ) ;
#13415=CARTESIAN_POINT ( 'NONE',  ( -42.49999999999999289, -38.78532556477446036, 90.66066734786068082 ) ) ;
#13461=ORIENTED_EDGE ( 'NONE', *, *, #34428, .T. ) ;
#13465=LINE ( 'NONE', #34590, #25091 ) ;
#13487=EDGE_CURVE ( 'NONE', #30439, #11413, #3539, .T. ) ;
#13493=EDGE_CURVE ( 'NONE', #8147, #26137, #6569, .T. ) ;
#13511=VERTEX_POINT ( 'NONE', #34313 ) ;
#13524=ADVANCED_FACE ( 'NONE', ( #12522 ), #24054, .T. ) ;
#13558=ORIENTED_EDGE ( 'NONE', *, *, #9162, .F. ) ;
#13609=EDGE_CURVE ( 'NONE', #793, #27859, #7292, .T. ) ;
#13612=ORIENTED_EDGE ( 'NONE', *, *, #24656, .F. ) ;
#13622=CARTESIAN_POINT ( 'NONE',  ( -21.15833593587365513, -24.48076211353301801, 67.99999999999991473 ) ) ;
#13628=DIRECTION ( 'NONE',  ( 0.000000000000000000, 0.8660254037844428154, -0.4999999999999929501 ) ) ;
#13638=ADVANCED_FACE ( 'NONE', ( #20602 ), #1540, .T. ) ;
#13689=ORIENTED_EDGE ( 'NONE', *, *, #34428, .F. ) ;
#13730=ADVANCED_FACE ( 'NONE', ( #18808 ), #21490, .T. ) ;
#13732=CARTESIAN_POINT ( 'NONE',  ( -42.49999999999999289, -16.18172400785637777, 71.02756813566458050 ) ) ;
#13745=EDGE_CURVE ( 'NONE', #21122, #6172, #11068, .T. ) ;
#13747=VECTOR ( 'NONE', #24418, 1000.000000000000000 ) ;
#13755=LINE ( 'NONE', #16425, #138 ) ;
#13757=FACE_OUTER_BOUND ( 'NONE', #33279, .T. ) ;
#13767=DIRECTION ( 'NONE',  ( -1.000000000000000000, 8.673617379883896189E-17, 1.502314598737167413E-16 ) ) ;
#13770=EDGE_CURVE ( 'NONE', #28824, #14767, #24396, .T. ) ;
#13771=ORIENTED_EDGE ( 'NONE', *, *, #29600, .T. ) ;
#13799=CIRCLE ( 'NONE', #18956, 14.00000000000000000 ) ;
#13809=CARTESIAN_POINT ( 'NONE',  ( -21.15833593587365513, -25.27980021920979326, 80.78589838486217900 ) ) ;
#13818=VERTEX_POINT ( 'NONE', #13415 ) ;
#13831=EDGE_LOOP ( 'NONE', ( #8107, #13991, #2957, #1107 ) ) ;
#13841=CARTESIAN_POINT ( 'NONE',  ( -34.49999999999998579, -27.48076211353304998, 70.99999999999988631 ) ) ;
#13843=COLOUR_RGB ( '', 0.40784314, 0.44705882, 0.49803922) ;
#13877=ORIENTED_EDGE ( 'NONE', *, *, #10637, .T. ) ;
#13882=DIRECTION ( 'NONE',  ( -1.000000000000000000, 0.000000000000000000, -0.000000000000000000 ) ) ;
#13956=AXIS2_PLACEMENT_3D ( 'NONE', #7243, #14984, #34806 ) ;
#13977=CARTESIAN_POINT ( 'NONE',  ( -21.15833593587365513, -20.27980021920970799, 72.12564434701783966 ) ) ;
#13991=ORIENTED_EDGE ( 'NONE', *, *, #6869, .T. ) ;
#14004=DIRECTION ( 'NONE',  ( -1.000000000000000000, -1.502314598737158292E-16, -8.673617379884052728E-17 ) ) ;
#14017=CARTESIAN_POINT ( 'NONE',  ( -34.49999999999998579, -25.98076211353322051, 84.99999999999992895 ) ) ;
#14028=ORIENTED_EDGE ( 'NONE', *, *, #24706, .F. ) ;
#14061=CARTESIAN_POINT ( 'NONE',  ( -21.15833593587365513, -13.10640646055107084, 90.70096189432331357 ) ) ;
#14066=DIRECTION ( 'NONE',  ( 0.000000000000000000, -1.000000000000000000, 0.000000000000000000 ) ) ;
#14069=VERTEX_POINT ( 'NONE', #484 ) ;
#14089=LINE ( 'NONE', #22191, #26465 ) ;
#14117=VERTEX_POINT ( 'NONE', #22263 ) ;
#14121=( NAMED_UNIT ( * ) SI_UNIT ( $, .STERADIAN. ) SOLID_ANGLE_UNIT ( ) );
#14172=EDGE_CURVE ( 'NONE', #13818, #13511, #4446, .T. ) ;
#14184=DIRECTION ( 'NONE',  ( -1.000000000000000000, -1.734723475976807094E-16, -0.000000000000000000 ) ) ;
#14188=PLANE ( 'NONE',  #6504 ) ;
#14212=VERTEX_POINT ( 'NONE', #12714 ) ;
#14215=AXIS2_PLACEMENT_3D ( 'NONE', #12987, #4726, #26682 ) ;
#14218=ORIENTED_EDGE ( 'NONE', *, *, #26936, .F. ) ;
#14219=ORIENTED_EDGE ( 'NONE', *, *, #16541, .F. ) ;
#14236=ORIENTED_EDGE ( 'NONE', *, *, #33243, .F. ) ;
#14257=CARTESIAN_POINT ( 'NONE',  ( -34.49999999999998579, -27.93100416606583991, 81.50764321173598148 ) ) ;
#14267=DIRECTION ( 'NONE',  ( 0.000000000000000000, 0.5000000000000031086, -0.8660254037844368202 ) ) ;
#14282=PLANE ( 'NONE',  #34359 ) ;
#14352=CARTESIAN_POINT ( 'NONE',  ( -42.49999999999999289, -13.17619866229204284, 90.66066734786082293 ) ) ;
#14359=DIRECTION ( 'NONE',  ( 0.000000000000000000, -1.000000000000000000, 0.000000000000000000 ) ) ;
#14365=DIRECTION ( 'NONE',  ( -1.000000000000000000, -1.817026393327835042E-30, 1.734723475976807094E-16 ) ) ;
#14366=ORIENTED_EDGE ( 'NONE', *, *, #9462, .T. ) ;
#14375=ORIENTED_EDGE ( 'NONE', *, *, #24318, .F. ) ;
#14450=EDGE_LOOP ( 'NONE', ( #33596, #9165, #20244, #16419 ) ) ;
#14458=( NAMED_UNIT ( * ) SI_UNIT ( $, .STERADIAN. ) SOLID_ANGLE_UNIT ( ) );
#14460=FACE_OUTER_BOUND ( 'NONE', #32636, .T. ) ;
#14464=ORIENTED_EDGE ( 'NONE', *, *, #22086, .T. ) ;
#14473=LINE ( 'NONE', #22758, #697 ) ;
#14487=DIRECTION ( 'NONE',  ( -0.000000000000000000, -0.2538061376417690140, -0.9672551082808337197 ) ) ;
#14529=LINE ( 'NONE', #28416, #23609 ) ;
#14575=ORIENTED_EDGE ( 'NONE', *, *, #11906, .T. ) ;
#14587=VECTOR ( 'NONE', #8455, 999.9999999999998863 ) ;
#14592=ORIENTED_EDGE ( 'NONE', *, *, #6035, .F. ) ;
#14608=EDGE_LOOP ( 'NONE', ( #1377, #3305, #17169, #11044 ) ) ;
#14614=VECTOR ( 'NONE', #29365, 1000.000000000000000 ) ;
#14622=CARTESIAN_POINT ( 'NONE',  ( -42.49999999999999289, -12.00833024919776371, 94.79903810567661537 ) ) ;
#14645=ORIENTED_EDGE ( 'NONE', *, *, #24984, .F. ) ;
#14664=DIRECTION ( 'NONE',  ( 0.000000000000000000, -1.000000000000000000, 0.000000000000000000 ) ) ;
#14684=EDGE_LOOP ( 'NONE', ( #3594, #35279, #13030, #24493 ) ) ;
#14687=DIRECTION ( 'NONE',  ( 0.000000000000000000, -1.067522139062650474E-15, -1.000000000000000000 ) ) ;
#14700=CARTESIAN_POINT ( 'NONE',  ( -34.50000000000001421, -12.00833024919776371, 94.79903810567661537 ) ) ;
#14746=CARTESIAN_POINT ( 'NONE',  ( -21.15833593587365513, -24.48076211353329157, 98.99999999999994316 ) ) ;
#14757=EDGE_CURVE ( 'NONE', #23698, #16800, #31989, .T. ) ;
#14767=VERTEX_POINT ( 'NONE', #14827 ) ;
#14827=CARTESIAN_POINT ( 'NONE',  ( -34.49999999999998579, -34.27980021920977549, 73.62564434701768334 ) ) ;
#14853=DIRECTION ( 'NONE',  ( 0.000000000000000000, -0.8660254037844350439, -0.5000000000000061062 ) ) ;
#14867=CARTESIAN_POINT ( 'NONE',  ( -34.49999999999998579, -25.99649394950417047, 81.00003093645244689 ) ) ;
#14901=LINE ( 'NONE', #31125, #289 ) ;
#14934=ORIENTED_EDGE ( 'NONE', *, *, #32762, .T. ) ;
#14942=EDGE_CURVE ( 'NONE', #10214, #13511, #13210, .T. ) ;
#14983=PLANE ( 'NONE',  #10246 ) ;
#14984=DIRECTION ( 'NONE',  ( -0.000000000000000000, -0.9659258262890674240, -0.2588190451025240701 ) ) ;
#15026=CARTESIAN_POINT ( 'NONE',  ( -34.49999999999998579, -22.68172400785658382, 87.71410161513770731 ) ) ;
#15028=LINE ( 'NONE', #1363, #30309 ) ;
#15036=PLANE ( 'NONE',  #24436 ) ;
#15048=CARTESIAN_POINT ( 'NONE',  ( -42.49999999999999289, -22.68172400785649501, 82.28589838486220742 ) ) ;
#15049=ORIENTED_EDGE ( 'NONE', *, *, #9326, .F. ) ;
#15061=CARTESIAN_POINT ( 'NONE',  ( -34.49999999999998579, -25.98076211353320986, 84.99999999999994316 ) ) ;
#15091=PLANE ( 'NONE',  #4233 ) ;
#15104=LINE ( 'NONE', #26113, #2701 ) ;
#15116=ORIENTED_EDGE ( 'NONE', *, *, #16794, .F. ) ;
#15124=ADVANCED_FACE ( 'NONE', ( #27427 ), #32820, .T. ) ;
#15135=ORIENTED_EDGE ( 'NONE', *, *, #20086, .F. ) ;
#15141=ORIENTED_EDGE ( 'NONE', *, *, #28401, .F. ) ;
#15168=CARTESIAN_POINT ( 'NONE',  ( -21.15833593587365513, -27.48076211353330578, 101.9999999999999432 ) ) ;
#15185=DIRECTION ( 'NONE',  ( -1.734723475976807094E-16, 0.5000000000000092149, -0.8660254037844333785 ) ) ;
#15186=LINE ( 'NONE', #20948, #30137 ) ;
#15215=AXIS2_PLACEMENT_3D ( 'NONE', #31198, #6526, #23459 ) ;
#15237=CARTESIAN_POINT ( 'NONE',  ( -34.49999999999998579, -37.28532556477433246, 76.74125644078564790 ) ) ;
#15259=ORIENTED_EDGE ( 'NONE', *, *, #16541, .T. ) ;
#15285=VERTEX_POINT ( 'NONE', #1470 ) ;
#15312=LINE ( 'NONE', #9925, #24208 ) ;
#15341=VECTOR ( 'NONE', #32679, 1000.000000000000000 ) ;
#15379=CARTESIAN_POINT ( 'NONE',  ( -34.49999999999998579, -25.98076211353322051, 84.99999999999992895 ) ) ;
#15425=DIRECTION ( 'NONE',  ( 1.000000000000000000, 1.734723475976807094E-16, 0.000000000000000000 ) ) ;
#15450=CARTESIAN_POINT ( 'NONE',  ( -34.49999999999998579, -31.64142946139417134, 97.80456345124110840 ) ) ;
#15565=LINE ( 'NONE', #5161, #24992 ) ;
#15629=VECTOR ( 'NONE', #24577, 1000.000000000000000 ) ;
#15632=LINE ( 'NONE', #21753, #19976 ) ;
#15646=VECTOR ( 'NONE', #26402, 1000.000000000000000 ) ;
#15651=ORIENTED_EDGE ( 'NONE', *, *, #7955, .F. ) ;
#15686=DIRECTION ( 'NONE',  ( 1.000000000000000000, 1.734723475976807094E-16, 0.000000000000000000 ) ) ;
#15687=VECTOR ( 'NONE', #7917, 1000.000000000000114 ) ;
#15689=CARTESIAN_POINT ( 'NONE',  ( -21.15833593587365513, -29.98076211353323828, 86.49999999999990052 ) ) ;
#15693=ORIENTED_EDGE ( 'NONE', *, *, #32762, .F. ) ;
#15753=EDGE_LOOP ( 'NONE', ( #21888, #20668, #10726, #29892 ) ) ;
#15802=EDGE_LOOP ( 'NONE', ( #21486, #2980, #13612, #14366 ) ) ;
#15803=DIRECTION ( 'NONE',  ( 0.000000000000000000, -1.000000000000000000, 1.067522139062650474E-15 ) ) ;
#15816=CARTESIAN_POINT ( 'NONE',  ( -34.49999999999998579, -25.27980021920989984, 89.21410161513769310 ) ) ;
#15848=VERTEX_POINT ( 'NONE', #5726 ) ;
#15873=VECTOR ( 'NONE', #23051, 1000.000000000000114 ) ;
#15893=ORIENTED_EDGE ( 'NONE', *, *, #21844, .T. ) ;
#15912=VECTOR ( 'NONE', #32907, 1000.000000000000000 ) ;
#15915=DIRECTION ( 'NONE',  ( 1.000000000000000000, 1.734723475976807094E-16, 0.000000000000000000 ) ) ;
#15917=DIRECTION ( 'NONE',  ( 0.000000000000000000, -0.8660254037844444808, 0.4999999999999898415 ) ) ;
#15926=ORIENTED_EDGE ( 'NONE', *, *, #2267, .F. ) ;
#15995=ADVANCED_FACE ( 'NONE', ( #28391 ), #6421, .T. ) ;
#16074=EDGE_CURVE ( 'NONE', #34282, #19124, #9678, .T. ) ;
#16087=CARTESIAN_POINT ( 'NONE',  ( -21.15833593587365513, -23.26666049839546702, 88.29903810567660116 ) ) ;
#16100=LINE ( 'NONE', #30167, #9632 ) ;
#16122=DIRECTION ( 'NONE',  ( -1.226634733346697831E-16, 0.2588190451025308425, -0.9659258262890655367 ) ) ;
#16123=DIRECTION ( 'NONE',  ( 0.000000000000000000, 0.7071067811865392461, 0.7071067811865557884 ) ) ;
#16131=CARTESIAN_POINT ( 'NONE',  ( -34.49999999999998579, -23.14406523420367634, 74.41330312067054820 ) ) ;
#16170=DIRECTION ( 'NONE',  ( 1.000000000000000000, 1.734723475976807094E-16, 0.000000000000000000 ) ) ;
#16181=VERTEX_POINT ( 'NONE', #24558 ) ;
#16267=EDGE_CURVE ( 'NONE', #25177, #12635, #24376, .T. ) ;
#16320=CARTESIAN_POINT ( 'NONE',  ( -34.49999999999998579, -14.67619866229190961, 76.74125644078588948 ) ) ;
#16335=ORIENTED_EDGE ( 'NONE', *, *, #31731, .F. ) ;
#16336=FACE_OUTER_BOUND ( 'NONE', #21986, .T. ) ;
#16401=ORIENTED_EDGE ( 'NONE', *, *, #14172, .F. ) ;
#16409=ORIENTED_EDGE ( 'NONE', *, *, #24490, .F. ) ;
#16419=ORIENTED_EDGE ( 'NONE', *, *, #11013, .F. ) ;
#16425=CARTESIAN_POINT ( 'NONE',  ( -42.49999999999999289, -26.68172400785662290, 89.21410161513769310 ) ) ;
#16429=FACE_OUTER_BOUND ( 'NONE', #19165, .T. ) ;
#16437=PLANE ( 'NONE',  #8277 ) ;
#16438=ORIENTED_EDGE ( 'NONE', *, *, #17748, .T. ) ;
#16441=CARTESIAN_POINT ( 'NONE',  ( -42.49999999999999289, -12.06135120645816272, 83.49999999999992895 ) ) ;
#16462=ORIENTED_EDGE ( 'NONE', *, *, #33430, .F. ) ;
#16474=EDGE_CURVE ( 'NONE', #26137, #19399, #22537, .T. ) ;
#16528=VECTOR ( 'NONE', #12589, 1000.000000000000114 ) ;
#16539=PLANE ( 'NONE',  #6894 ) ;
#16541=EDGE_CURVE ( 'NONE', #6172, #3694, #16610, .T. ) ;
#16545=LINE ( 'NONE', #8087, #18150 ) ;
#16610=CIRCLE ( 'NONE', #5126, 14.00000000000000000 ) ;
#16665=LINE ( 'NONE', #642, #20381 ) ;
#16672=PLANE ( 'NONE',  #30847 ) ;
#16696=LINE ( 'NONE', #28229, #27610 ) ;
#16723=EDGE_CURVE ( 'NONE', #3468, #11685, #10304, .T. ) ;
#16733=EDGE_CURVE ( 'NONE', #2158, #32986, #6739, .T. ) ;
#16736=ORIENTED_EDGE ( 'NONE', *, *, #24272, .F. ) ;
#16758=DIRECTION ( 'NONE',  ( -1.000000000000000000, 0.000000000000000000, -0.000000000000000000 ) ) ;
#16794=EDGE_CURVE ( 'NONE', #10255, #9519, #10511, .T. ) ;
#16800=VERTEX_POINT ( 'NONE', #24736 ) ;
#16821=DIRECTION ( 'NONE',  ( -1.000000000000000000, 1.734723475976807094E-16, 0.000000000000000000 ) ) ;
#16842=DIRECTION ( 'NONE',  ( -1.734723475976806848E-16, -0.8660254037844410391, 0.4999999999999958367 ) ) ;
#16867=EDGE_LOOP ( 'NONE', ( #15651, #10100, #30250, #4847 ) ) ;
#16905=ORIENTED_EDGE ( 'NONE', *, *, #2302, .F. ) ;
#16954=VECTOR ( 'NONE', #23548, 1000.000000000000000 ) ;
#16994=LINE ( 'NONE', #273, #22355 ) ;
#17008=CARTESIAN_POINT ( 'NONE',  ( -34.49999999999998579, -39.90017302060827831, 86.49999999999991473 ) ) ;
#17011=LINE ( 'NONE', #1011, #3003 ) ;
#17030=VERTEX_POINT ( 'NONE', #25081 ) ;
#17037=VECTOR ( 'NONE', #11453, 1000.000000000000114 ) ;
#17039=AXIS2_PLACEMENT_3D ( 'NONE', #33516, #746, #24722 ) ;
#17057=CARTESIAN_POINT ( 'NONE',  ( -34.49999999999998579, -25.98076211353322051, 84.99999999999992895 ) ) ;
#17089=EDGE_CURVE ( 'NONE', #14069, #7962, #7052, .T. ) ;
#17095=CARTESIAN_POINT ( 'NONE',  ( -34.49999999999998579, -20.32009476567217376, 72.19543654875880634 ) ) ;
#17108=CARTESIAN_POINT ( 'NONE',  ( -34.49999999999998579, -26.38406014851792847, 79.52301627764165914 ) ) ;
#17119=DIRECTION ( 'NONE',  ( -1.000000000000000000, -1.734723475976807094E-16, -0.000000000000000000 ) ) ;
#17121=EDGE_CURVE ( 'NONE', #2498, #9312, #25855, .T. ) ;
#17135=VERTEX_POINT ( 'NONE', #4567 ) ;
#17146=CARTESIAN_POINT ( 'NONE',  ( -42.49999999999999289, -39.95319397786859383, 75.20096189432314304 ) ) ;
#17148=CARTESIAN_POINT ( 'NONE',  ( -42.49999999999999289, -25.98076211353322051, 84.99999999999992895 ) ) ;
#17159=ORIENTED_EDGE ( 'NONE', *, *, #16474, .F. ) ;
#17169=ORIENTED_EDGE ( 'NONE', *, *, #11906, .F. ) ;
#17204=LINE ( 'NONE', #11293, #32698 ) ;
#17239=ORIENTED_EDGE ( 'NONE', *, *, #22902, .T. ) ;
#17247=ORIENTED_EDGE ( 'NONE', *, *, #24071, .T. ) ;
#17251=DIRECTION ( 'NONE',  ( 1.000000000000000000, 1.734723475976807094E-16, 0.000000000000000000 ) ) ;
#17268=STYLED_ITEM ( 'NONE', ( #11434 ), #17621 ) ;
#17306=ORIENTED_EDGE ( 'NONE', *, *, #4568, .F. ) ;
#17367=FACE_OUTER_BOUND ( 'NONE', #7633, .T. ) ;
#17395=FACE_OUTER_BOUND ( 'NONE', #13313, .T. ) ;
#17415=VECTOR ( 'NONE', #9598, 1000.000000000000000 ) ;
#17466=DIRECTION ( 'NONE',  ( 1.000000000000000000, 1.734723475976807094E-16, 0.000000000000000000 ) ) ;
#17490=ADVANCED_FACE ( 'NONE', ( #16336 ), #2700, .T. ) ;
#17505=DIRECTION ( 'NONE',  ( 1.000000000000000000, 1.734723475976807094E-16, 0.000000000000000000 ) ) ;
#17507=VECTOR ( 'NONE', #20018, 1000.000000000000114 ) ;
#17512=LINE ( 'NONE', #4044, #1772 ) ;
#17546=CARTESIAN_POINT ( 'NONE',  ( -34.49999999999998579, -21.98076211353320630, 83.49999999999994316 ) ) ;
#17572=ORIENTED_EDGE ( 'NONE', *, *, #27527, .T. ) ;
#17578=DIRECTION ( 'NONE',  ( -1.000000000000000000, -1.734723475976807094E-16, -0.000000000000000000 ) ) ;
#17582=FACE_OUTER_BOUND ( 'NONE', #20082, .T. ) ;
#17587=FACE_OUTER_BOUND ( 'NONE', #33933, .T. ) ;
#17614=EDGE_CURVE ( 'NONE', #23698, #2158, #16696, .T. ) ;
#17621=ADVANCED_BREP_SHAPE_REPRESENTATION ( '', ( #34526, #21307 ), #24207 ) ;
#17640=ORIENTED_EDGE ( 'NONE', *, *, #32146, .F. ) ;
#17648=VECTOR ( 'NONE', #2977, 1000.000000000000000 ) ;
#17695=EDGE_LOOP ( 'NONE', ( #26125, #23707, #30198, #32484 ) ) ;
#17699=CARTESIAN_POINT ( 'NONE',  ( -42.49999999999999289, -25.27980021920989984, 89.21410161513770731 ) ) ;
#17710=ORIENTED_EDGE ( 'NONE', *, *, #9466, .F. ) ;
#17734=CARTESIAN_POINT ( 'NONE',  ( -42.49999999999999289, -42.98076211353323828, 83.49999999999991473 ) ) ;
#17743=ORIENTED_EDGE ( 'NONE', *, *, #25314, .T. ) ;
#17746=ORIENTED_EDGE ( 'NONE', *, *, #10861, .T. ) ;
#17748=EDGE_CURVE ( 'NONE', #19124, #27521, #17761, .T. ) ;
#17749=VERTEX_POINT ( 'NONE', #14700 ) ;
#17754=LINE ( 'NONE', #15048, #12745 ) ;
#17761=LINE ( 'NONE', #23172, #30324 ) ;
#17782=VERTEX_POINT ( 'NONE', #23347 ) ;
#17785=VERTEX_POINT ( 'NONE', #9842 ) ;
#17798=CARTESIAN_POINT ( 'NONE',  ( -21.15833593587365513, -21.76666049839542438, 84.29903810567665801 ) ) ;
#17865=MECHANICAL_DESIGN_GEOMETRIC_PRESENTATION_REPRESENTATION('',(#17268),#2383);
#17880=PLANE ( 'NONE',  #29535 ) ;
#17909=LINE ( 'NONE', #15026, #1448 ) ;
#17921=ORIENTED_EDGE ( 'NONE', *, *, #34184, .T. ) ;
#17938=VECTOR ( 'NONE', #31806, 999.9999999999998863 ) ;
#17947=DIRECTION ( 'NONE',  ( -1.000000000000000000, 1.502314598737152375E-16, 8.673617379884158732E-17 ) ) ;
#17958=ORIENTED_EDGE ( 'NONE', *, *, #34999, .T. ) ;
#17996=VERTEX_POINT ( 'NONE', #12737 ) ;
#17999=CARTESIAN_POINT ( 'NONE',  ( -42.49999999999999289, -27.48076211353304998, 70.99999999999988631 ) ) ;
#18053=ORIENTED_EDGE ( 'NONE', *, *, #13493, .T. ) ;
#18087=VECTOR ( 'NONE', #2143, 1000.000000000000000 ) ;
#18101=ORIENTED_EDGE ( 'NONE', *, *, #1745, .F. ) ;
#18114=VECTOR ( 'NONE', #25324, 1000.000000000000000 ) ;
#18115=CYLINDRICAL_SURFACE ( 'NONE', #23110, 13.99999999999999822 ) ;
#18124=DIRECTION ( 'NONE',  ( 1.000000000000000000, 1.734723475976807094E-16, 0.000000000000000000 ) ) ;
#18127=PLANE ( 'NONE',  #10781 ) ;
#18150=VECTOR ( 'NONE', #14365, 1000.000000000000000 ) ;
#18177=LINE ( 'NONE', #34042, #33017 ) ;
#18222=EDGE_LOOP ( 'NONE', ( #33359, #23795, #17921, #16335 ) ) ;
#18233=AXIS2_PLACEMENT_3D ( 'NONE', #21320, #4086, #7469 ) ;
#18247=ORIENTED_EDGE ( 'NONE', *, *, #31210, .F. ) ;
#18274=EDGE_CURVE ( 'NONE', #11413, #21432, #1350, .T. ) ;
#18292=DIRECTION ( 'NONE',  ( 1.000000000000000000, 0.000000000000000000, 0.000000000000000000 ) ) ;
#18296=DIRECTION ( 'NONE',  ( 0.000000000000000000, -1.000000000000000000, -2.423959199780483078E-15 ) ) ;
#18298=ORIENTED_EDGE ( 'NONE', *, *, #22659, .F. ) ;
#18312=EDGE_CURVE ( 'NONE', #27521, #14212, #29841, .T. ) ;
#18357=LINE ( 'NONE', #4336, #3340 ) ;
#18370=CARTESIAN_POINT ( 'NONE',  ( -42.49999999999999289, -20.27980021920970799, 72.12564434701783966 ) ) ;
#18424=ORIENTED_EDGE ( 'NONE', *, *, #9420, .T. ) ;
#18429=CARTESIAN_POINT ( 'NONE',  ( -42.49999999999999289, -18.77980021920990694, 100.4724318643354053 ) ) ;
#18434=VECTOR ( 'NONE', #31031, 1000.000000000000000 ) ;
#18460=CARTESIAN_POINT ( 'NONE',  ( -34.49999999999998579, -37.35511776651544125, 93.29903810567650169 ) ) ;
#18468=EDGE_CURVE ( 'NONE', #27933, #22358, #8116, .T. ) ;
#18501=ORIENTED_EDGE ( 'NONE', *, *, #8882, .F. ) ;
#18564=ORIENTED_EDGE ( 'NONE', *, *, #22499, .T. ) ;
#18570=VECTOR ( 'NONE', #4055, 1000.000000000000000 ) ;
#18587=ORIENTED_EDGE ( 'NONE', *, *, #6035, .T. ) ;
#18592=DIRECTION ( 'NONE',  ( -1.000000000000000000, -1.734723475976807094E-16, -0.000000000000000000 ) ) ;
#18623=CARTESIAN_POINT ( 'NONE',  ( -34.49999999999998579, -25.98076211353320986, 84.99999999999994316 ) ) ;
#18632=DIRECTION ( 'NONE',  ( -1.000000000000000000, -1.734723475976807094E-16, -0.000000000000000000 ) ) ;
#18640=LINE ( 'NONE', #24768, #26453 ) ;
#18645=( NAMED_UNIT ( * ) PLANE_ANGLE_UNIT ( ) SI_UNIT ( $, .RADIAN. ) );
#18652=VERTEX_POINT ( 'NONE', #17095 ) ;
#18668=ORIENTED_EDGE ( 'NONE', *, *, #1665, .T. ) ;
#18682=CARTESIAN_POINT ( 'NONE',  ( -21.15833593587365513, -27.48076211353326670, 88.99999999999994316 ) ) ;
#18808=FACE_OUTER_BOUND ( 'NONE', #25479, .T. ) ;
#18872=ORIENTED_EDGE ( 'NONE', *, *, #2748, .T. ) ;
#18895=ORIENTED_EDGE ( 'NONE', *, *, #9462, .F. ) ;
#18898=EDGE_CURVE ( 'NONE', #5903, #15285, #15632, .T. ) ;
#18901=LINE ( 'NONE', #24142, #15687 ) ;
#18956=AXIS2_PLACEMENT_3D ( 'NONE', #29525, #4860, #26821 ) ;
#18966=CARTESIAN_POINT ( 'NONE',  ( -34.49999999999998579, -24.48076211353314591, 80.99999999999991473 ) ) ;
#18969=FACE_OUTER_BOUND ( 'NONE', #15753, .T. ) ;
#18981=DIRECTION ( 'NONE',  ( -1.734723475976807094E-16, 0.8660254037844385966, 0.5000000000000001110 ) ) ;
#19078=ORIENTED_EDGE ( 'NONE', *, *, #2520, .T. ) ;
#19083=PLANE ( 'NONE',  #14215 ) ;
#19112=AXIS2_PLACEMENT_3D ( 'NONE', #6531, #17505, #3144 ) ;
#19124=VERTEX_POINT ( 'NONE', #23703 ) ;
#19154=EDGE_CURVE ( 'NONE', #8803, #27165, #12906, .T. ) ;
#19165=EDGE_LOOP ( 'NONE', ( #18895, #14375, #18424, #33909 ) ) ;
#19175=FILL_AREA_STYLE_COLOUR ( '', #13843 ) ;
#19176=VERTEX_POINT ( 'NONE', #35405 ) ;
#19196=CARTESIAN_POINT ( 'NONE',  ( -21.15833593587365513, -30.19486372867100954, 85.70096189432321410 ) ) ;
#19205=EDGE_LOOP ( 'NONE', ( #11124, #15693, #29545, #31136 ) ) ;
#19220=DIRECTION ( 'NONE',  ( -1.000000000000000000, 1.502314598737164455E-16, -8.673617379883947958E-17 ) ) ;
#19235=FACE_OUTER_BOUND ( 'NONE', #21544, .T. ) ;
#19236=EDGE_CURVE ( 'NONE', #15285, #17135, #19348, .T. ) ;
#19252=DIRECTION ( 'NONE',  ( 1.000000000000000000, 1.734723475976807094E-16, 0.000000000000000000 ) ) ;
#19278=VERTEX_POINT ( 'NONE', #11091 ) ;
#19320=ORIENTED_EDGE ( 'NONE', *, *, #14942, .F. ) ;
#19327=DIRECTION ( 'NONE',  ( 1.000000000000000000, 0.000000000000000000, 0.000000000000000000 ) ) ;
#19334=EDGE_CURVE ( 'NONE', #24482, #8803, #35064, .T. ) ;
#19335=VECTOR ( 'NONE', #26721, 1000.000000000000000 ) ;
#19348=LINE ( 'NONE', #30177, #31551 ) ;
#19350=VECTOR ( 'NONE', #12427, 1000.000000000000000 ) ;
#19386=EDGE_CURVE ( 'NONE', #34028, #32406, #16994, .T. ) ;
#19391=AXIS2_PLACEMENT_3D ( 'NONE', #16087, #27466, #8002 ) ;
#19399=VERTEX_POINT ( 'NONE', #28180 ) ;
#19416=DIRECTION ( 'NONE',  ( 0.000000000000000000, -0.8660254037844385966, -0.5000000000000001110 ) ) ;
#19430=CARTESIAN_POINT ( 'NONE',  ( -42.49999999999999289, -27.48076211353330578, 101.9999999999999432 ) ) ;
#19446=EDGE_CURVE ( 'NONE', #9156, #28748, #25480, .T. ) ;
#19463=AXIS2_PLACEMENT_3D ( 'NONE', #22762, #11785, #33766 ) ;
#19485=DIRECTION ( 'NONE',  ( 1.226634733346697831E-16, 0.9659258262890698665, -0.2588190451025151884 ) ) ;
#19501=CARTESIAN_POINT ( 'NONE',  ( 75.00000000000001421, -25.99649394950417047, 81.00003093645244689 ) ) ;
#19542=AXIS2_PLACEMENT_3D ( 'NONE', #7454, #23851, #13232 ) ;
#19545=CARTESIAN_POINT ( 'NONE',  ( -34.49999999999998579, -25.01350700525237514, 84.74619386235816876 ) ) ;
#19570=CARTESIAN_POINT ( 'NONE',  ( -34.49999999999998579, -25.98076211353322051, 84.99999999999992895 ) ) ;
#19616=FACE_OUTER_BOUND ( 'NONE', #16867, .T. ) ;
#19618=CARTESIAN_POINT ( 'NONE',  ( -34.49999999999998579, -12.06135120645816627, 83.49999999999992895 ) ) ;
#19652=CIRCLE ( 'NONE', #21955, 14.00000000000000000 ) ;
#19677=VERTEX_POINT ( 'NONE', #8032 ) ;
#19685=ORIENTED_EDGE ( 'NONE', *, *, #20121, .T. ) ;
#19707=PLANE ( 'NONE',  #21639 ) ;
#19709=ORIENTED_EDGE ( 'NONE', *, *, #30788, .T. ) ;
#19718=AXIS2_PLACEMENT_3D ( 'NONE', #24882, #11192, #22515 ) ;
#19732=CARTESIAN_POINT ( 'NONE',  ( -42.49999999999999289, -12.00833024919776371, 94.79903810567661537 ) ) ;
#19737=DIRECTION ( 'NONE',  ( 0.000000000000000000, -1.000000000000000000, 0.000000000000000000 ) ) ;
#19765=FACE_OUTER_BOUND ( 'NONE', #9039, .T. ) ;
#19772=ORIENTED_EDGE ( 'NONE', *, *, #23228, .T. ) ;
#19780=CARTESIAN_POINT ( 'NONE',  ( -21.15833593587365513, -16.18172400785637777, 71.02756813566458050 ) ) ;
#19811=ORIENTED_EDGE ( 'NONE', *, *, #13745, .F. ) ;
#19845=CARTESIAN_POINT ( 'NONE',  ( -42.49999999999999289, -37.28532556477433246, 76.74125644078564790 ) ) ;
#19847=FACE_OUTER_BOUND ( 'NONE', #30265, .T. ) ;
#19858=VECTOR ( 'NONE', #28417, 1000.000000000000000 ) ;
#19945=DIRECTION ( 'NONE',  ( 0.000000000000000000, -1.000000000000000000, 0.000000000000000000 ) ) ;
#19976=VECTOR ( 'NONE', #32748, 1000.000000000000000 ) ;
#19993=ORIENTED_EDGE ( 'NONE', *, *, #10425, .T. ) ;
#19996=CARTESIAN_POINT ( 'NONE',  ( -42.49999999999999289, -35.77980021920998155, 98.97243186433534845 ) ) ;
#20016=UNCERTAINTY_MEASURE_WITH_UNIT (LENGTH_MEASURE( 1.000000000000000082E-05 ), #33391, 'distance_accuracy_value', 'NONE');
#20018=DIRECTION ( 'NONE',  ( 1.226634733346698078E-16, -0.2588190451025185190, -0.9659258262890689783 ) ) ;
#20026=LINE ( 'NONE', #17699, #18434 ) ;
#20032=EDGE_CURVE ( 'NONE', #21122, #29583, #25899, .T. ) ;
#20034=VECTOR ( 'NONE', #33011, 1000.000000000000000 ) ;
#20074=ORIENTED_EDGE ( 'NONE', *, *, #26001, .F. ) ;
#20082=EDGE_LOOP ( 'NONE', ( #11772, #35190, #21514, #27747 ) ) ;
#20086=EDGE_CURVE ( 'NONE', #17996, #15848, #26561, .T. ) ;
#20121=EDGE_CURVE ( 'NONE', #27197, #35019, #7625, .T. ) ;
#20194=CARTESIAN_POINT ( 'NONE',  ( -34.50000000000001421, -33.18172400785640264, 69.52756813566438154 ) ) ;
#20199=ADVANCED_FACE ( 'NONE', ( #16429 ), #10696, .T. ) ;
#20210=ORIENTED_EDGE ( 'NONE', *, *, #22684, .T. ) ;
#20238=CARTESIAN_POINT ( 'NONE',  ( -34.49999999999998579, -26.94801722181404102, 85.25380613764170334 ) ) ;
#20244=ORIENTED_EDGE ( 'NONE', *, *, #19386, .T. ) ;
#20278=ADVANCED_FACE ( 'NONE', ( #18969 ), #21845, .F. ) ;
#20282=CYLINDRICAL_SURFACE ( 'NONE', #20491, 13.99999999999999822 ) ;
#20289=ADVANCED_FACE ( 'NONE', ( #13757 ), #11224, .F. ) ;
#20292=EDGE_CURVE ( 'NONE', #13511, #29087, #14089, .T. ) ;
#20310=CIRCLE ( 'NONE', #29558, 14.00000000000000000 ) ;
#20366=CARTESIAN_POINT ( 'NONE',  ( -42.49999999999999289, -25.98076211353320986, 84.99999999999994316 ) ) ;
#20376=DIRECTION ( 'NONE',  ( -1.000000000000000000, 0.000000000000000000, -0.000000000000000000 ) ) ;
#20381=VECTOR ( 'NONE', #11620, 1000.000000000000000 ) ;
#20383=CARTESIAN_POINT ( 'NONE',  ( -34.49999999999998579, -12.06135120645816983, 86.49999999999994316 ) ) ;
#20412=DIRECTION ( 'NONE',  ( 0.000000000000000000, 0.4999999999999898415, 0.8660254037844444808 ) ) ;
#20429=ORIENTED_EDGE ( 'NONE', *, *, #1133, .F. ) ;
#20485=ADVANCED_FACE ( 'NONE', ( #3665 ), #33898, .T. ) ;
#20491=AXIS2_PLACEMENT_3D ( 'NONE', #17057, #3755, #14359 ) ;
#20503=AXIS2_PLACEMENT_3D ( 'NONE', #15379, #32318, #4259 ) ;
#20523=VECTOR ( 'NONE', #27843, 1000.000000000000000 ) ;
#20546=VERTEX_POINT ( 'NONE', #33449 ) ;
#20576=ADVANCED_FACE ( 'NONE', ( #17582 ), #28233, .T. ) ;
#20602=FACE_OUTER_BOUND ( 'NONE', #34267, .T. ) ;
#20633=CARTESIAN_POINT ( 'NONE',  ( -34.49999999999998579, -24.48076211353329157, 98.99999999999994316 ) ) ;
#20642=CARTESIAN_POINT ( 'NONE',  ( -42.49999999999999289, -24.48076211353329157, 98.99999999999994316 ) ) ;
#20668=ORIENTED_EDGE ( 'NONE', *, *, #13770, .T. ) ;
#20669=ORIENTED_EDGE ( 'NONE', *, *, #5513, .F. ) ;
#20705=VECTOR ( 'NONE', #23360, 1000.000000000000000 ) ;
#20715=ORIENTED_EDGE ( 'NONE', *, *, #2219, .T. ) ;
#20731=DIRECTION ( 'NONE',  ( -0.000000000000000000, -0.2538061376417690140, -0.9672551082808337197 ) ) ;
#20735=VECTOR ( 'NONE', #18592, 1000.000000000000000 ) ;
#20736=CARTESIAN_POINT ( 'NONE',  ( -34.49999999999998579, -17.72201855431888973, 73.69543654875883476 ) ) ;
#20746=EDGE_CURVE ( 'NONE', #21074, #4350, #26549, .T. ) ;
#20787=ORIENTED_EDGE ( 'NONE', *, *, #30517, .F. ) ;
#20789=CARTESIAN_POINT ( 'NONE',  ( -42.49999999999999289, -20.32009476567218798, 72.19543654875880634 ) ) ;
#20794=CARTESIAN_POINT ( 'NONE',  ( -34.49999999999998579, -38.78532556477437510, 79.33933265213894970 ) ) ;
#20799=CARTESIAN_POINT ( 'NONE',  ( -42.49999999999999289, -16.18172400785637777, 71.02756813566458050 ) ) ;
#20830=CARTESIAN_POINT ( 'NONE',  ( -42.49999999999997158, -25.99649394950417047, 81.00003093645244689 ) ) ;
#20834=VERTEX_POINT ( 'NONE', #20633 ) ;
#20878=ORIENTED_EDGE ( 'NONE', *, *, #4681, .T. ) ;
#20898=EDGE_CURVE ( 'NONE', #19399, #26771, #21353, .T. ) ;
#20905=DIRECTION ( 'NONE',  ( 0.000000000000000000, 1.000000000000000000, 0.000000000000000000 ) ) ;
#20909=ORIENTED_EDGE ( 'NONE', *, *, #7274, .F. ) ;
#20912=FACE_OUTER_BOUND ( 'NONE', #376, .T. ) ;
#20935=AXIS2_PLACEMENT_3D ( 'NONE', #24281, #33427, #11633 ) ;
#20945=ADVANCED_FACE ( 'NONE', ( #8379 ), #33063, .F. ) ;
#20948=CARTESIAN_POINT ( 'NONE',  ( -42.49999999999999289, -21.98076211353320630, 83.49999999999994316 ) ) ;
#20954=CARTESIAN_POINT ( 'NONE',  ( -34.49999999999998579, -25.98076211353322051, 84.99999999999992895 ) ) ;
#20975=CIRCLE ( 'NONE', #26161, 14.00000000000000000 ) ;
#20977=ORIENTED_EDGE ( 'NONE', *, *, #7479, .F. ) ;
#21015=PLANE ( 'NONE',  #20935 ) ;
#21039=LINE ( 'NONE', #2706, #28953 ) ;
#21048=CARTESIAN_POINT ( 'NONE',  ( -34.49999999999998579, -29.27980021920993536, 87.71410161513767889 ) ) ;
#21074=VERTEX_POINT ( 'NONE', #33239 ) ;
#21122=VERTEX_POINT ( 'NONE', #28192 ) ;
#21150=PLANE ( 'NONE',  #20503 ) ;
#21155=DIRECTION ( 'NONE',  ( 1.000000000000000000, 1.734723475976807094E-16, 0.000000000000000000 ) ) ;
#21176=ORIENTED_EDGE ( 'NONE', *, *, #1745, .T. ) ;
#21206=EDGE_LOOP ( 'NONE', ( #34982, #1771, #22344, #25079 ) ) ;
#21229=DIRECTION ( 'NONE',  ( 0.000000000000000000, -1.000000000000000000, 1.067522139062650474E-15 ) ) ;
#21240=ORIENTED_EDGE ( 'NONE', *, *, #13487, .F. ) ;
#21248=CARTESIAN_POINT ( 'NONE',  ( -42.49999999999999289, -25.98076211353322051, 84.99999999999992895 ) ) ;
#21274=EDGE_CURVE ( 'NONE', #18652, #223, #4076, .T. ) ;
#21290=CARTESIAN_POINT ( 'NONE',  ( -42.49999999999999289, -8.980762113533206303, 86.49999999999994316 ) ) ;
#21307=AXIS2_PLACEMENT_3D ( 'NONE', #26589, #12725, #18292 ) ;
#21320=CARTESIAN_POINT ( 'NONE',  ( -34.49999999999998579, -26.94801722181404102, 85.25380613764170334 ) ) ;
#21353=LINE ( 'NONE', #24613, #29988 ) ;
#21363=LINE ( 'NONE', #12567, #12472 ) ;
#21372=DIRECTION ( 'NONE',  ( -1.000000000000000000, -1.734723475976807094E-16, -0.000000000000000000 ) ) ;
#21396=ORIENTED_EDGE ( 'NONE', *, *, #20032, .T. ) ;
#21432=VERTEX_POINT ( 'NONE', #35201 ) ;
#21433=ORIENTED_EDGE ( 'NONE', *, *, #33432, .F. ) ;
#21470=ORIENTED_EDGE ( 'NONE', *, *, #24985, .T. ) ;
#21478=VECTOR ( 'NONE', #4784, 1000.000000000000000 ) ;
#21486=ORIENTED_EDGE ( 'NONE', *, *, #31089, .T. ) ;
#21490=PLANE ( 'NONE',  #19391 ) ;
#21507=( LENGTH_UNIT ( ) NAMED_UNIT ( * ) SI_UNIT ( .MILLI., .METRE. ) );
#21514=ORIENTED_EDGE ( 'NONE', *, *, #17614, .T. ) ;
#21544=EDGE_LOOP ( 'NONE', ( #4360, #22967, #8394, #17239 ) ) ;
#21587=CIRCLE ( 'NONE', #2065, 14.00000000000000000 ) ;
#21619=VECTOR ( 'NONE', #9455, 1000.000000000000000 ) ;
#21621=CARTESIAN_POINT ( 'NONE',  ( -34.49999999999998579, -25.98076211353322051, 84.99999999999992895 ) ) ;
#21622=ORIENTED_EDGE ( 'NONE', *, *, #5727, .F. ) ;
#21639=AXIS2_PLACEMENT_3D ( 'NONE', #13809, #32718, #24796 ) ;
#21642=LINE ( 'NONE', #21290, #19335 ) ;
#21656=CARTESIAN_POINT ( 'NONE',  ( -42.49999999999999289, -24.48076211353314591, 80.99999999999991473 ) ) ;
#21679=CARTESIAN_POINT ( 'NONE',  ( -34.49999999999998579, -27.48076211353329157, 98.91941090707497608 ) ) ;
#21753=CARTESIAN_POINT ( 'NONE',  ( -42.49999999999999289, -42.98076211353323828, 83.49999999999991473 ) ) ;
#21768=VECTOR ( 'NONE', #16821, 1000.000000000000000 ) ;
#21784=ORIENTED_EDGE ( 'NONE', *, *, #3953, .F. ) ;
#21810=EDGE_CURVE ( 'NONE', #14212, #31835, #2655, .T. ) ;
#21826=CARTESIAN_POINT ( 'NONE',  ( -42.49999999999999289, -13.10640646055107084, 90.70096189432331357 ) ) ;
#21844=EDGE_CURVE ( 'NONE', #34282, #14117, #1861, .T. ) ;
#21845=PLANE ( 'NONE',  #2346 ) ;
#21888=ORIENTED_EDGE ( 'NONE', *, *, #7479, .T. ) ;
#21901=PLANE ( 'NONE',  #874 ) ;
#21926=CARTESIAN_POINT ( 'NONE',  ( -34.49999999999998579, -25.98076211353322051, 84.99999999999992895 ) ) ;
#21935=CARTESIAN_POINT ( 'NONE',  ( -42.49999999999999289, -26.38406014851792847, 79.52301627764165914 ) ) ;
#21955=AXIS2_PLACEMENT_3D ( 'NONE', #31231, #34116, #6554 ) ;
#21976=DIRECTION ( 'NONE',  ( 0.000000000000000000, 0.9659258262890656477, 0.2588190451025308425 ) ) ;
#21986=EDGE_LOOP ( 'NONE', ( #1118, #2720, #11000, #22690 ) ) ;
#22050=CARTESIAN_POINT ( 'NONE',  ( -42.49999999999999289, -24.48076211353328802, 98.91941090707499029 ) ) ;
#22058=ORIENTED_EDGE ( 'NONE', *, *, #24272, .T. ) ;
#22086=EDGE_CURVE ( 'NONE', #9715, #2578, #30977, .T. ) ;
#22119=ORIENTED_EDGE ( 'NONE', *, *, #22902, .F. ) ;
#22136=DIRECTION ( 'NONE',  ( 0.000000000000000000, 1.000000000000000000, 0.000000000000000000 ) ) ;
#22137=DIRECTION ( 'NONE',  ( -1.000000000000000000, 0.000000000000000000, 0.000000000000000000 ) ) ;
#22151=VECTOR ( 'NONE', #16842, 1000.000000000000114 ) ;
#22181=LINE ( 'NONE', #19996, #9522 ) ;
#22182=ORIENTED_EDGE ( 'NONE', *, *, #33002, .T. ) ;
#22191=CARTESIAN_POINT ( 'NONE',  ( -42.49999999999999289, -41.45319397786874305, 92.20096189432314304 ) ) ;
#22231=CARTESIAN_POINT ( 'NONE',  ( -34.49999999999998579, -39.90017302060827831, 83.49999999999991473 ) ) ;
#22254=DIRECTION ( 'NONE',  ( -1.734723475976807094E-16, 1.000000000000000000, 0.000000000000000000 ) ) ;
#22263=CARTESIAN_POINT ( 'NONE',  ( -34.49999999999998579, -26.38406014851792847, 79.52301627764165914 ) ) ;
#22271=EDGE_CURVE ( 'NONE', #30700, #32761, #1445, .T. ) ;
#22294=CARTESIAN_POINT ( 'NONE',  ( -42.49999999999999289, -27.48076211353305354, 71.08058909292485339 ) ) ;
#22298=ORIENTED_EDGE ( 'NONE', *, *, #20292, .T. ) ;
#22311=ORIENTED_EDGE ( 'NONE', *, *, #26677, .F. ) ;
#22315=ORIENTED_EDGE ( 'NONE', *, *, #5799, .F. ) ;
#22344=ORIENTED_EDGE ( 'NONE', *, *, #230, .F. ) ;
#22349=ORIENTED_EDGE ( 'NONE', *, *, #11021, .T. ) ;
#22355=VECTOR ( 'NONE', #11779, 1000.000000000000000 ) ;
#22358=VERTEX_POINT ( 'NONE', #26835 ) ;
#22393=CARTESIAN_POINT ( 'NONE',  ( -42.49999999999999289, -25.98076211353322051, 84.99999999999992895 ) ) ;
#22421=DIRECTION ( 'NONE',  ( 0.000000000000000000, 0.8660254037844410391, -0.4999999999999958367 ) ) ;
#22438=CIRCLE ( 'NONE', #28188, 14.00000000000000000 ) ;
#22445=ORIENTED_EDGE ( 'NONE', *, *, #5805, .T. ) ;
#22483=ADVANCED_FACE ( 'NONE', ( #17367 ), #6049, .F. ) ;
#22493=DIRECTION ( 'NONE',  ( 0.000000000000000000, 9.406921877466749789E-15, -1.000000000000000000 ) ) ;
#22499=EDGE_CURVE ( 'NONE', #29247, #24192, #17011, .T. ) ;
#22515=DIRECTION ( 'NONE',  ( 0.000000000000000000, 1.000000000000000000, 0.000000000000000000 ) ) ;
#22537=LINE ( 'NONE', #8858, #30378 ) ;
#22559=DIRECTION ( 'NONE',  ( 0.000000000000000000, 1.000000000000000000, 9.406921877466749789E-15 ) ) ;
#22587=FACE_OUTER_BOUND ( 'NONE', #23448, .T. ) ;
#22648=CARTESIAN_POINT ( 'NONE',  ( -21.15833593587365513, -39.95319397786859383, 75.20096189432314304 ) ) ;
#22659=EDGE_CURVE ( 'NONE', #19278, #5903, #2089, .T. ) ;
#22671=DIRECTION ( 'NONE',  ( -1.000000000000000000, 0.000000000000000000, 0.000000000000000000 ) ) ;
#22684=EDGE_CURVE ( 'NONE', #30439, #31835, #2275, .T. ) ;
#22690=ORIENTED_EDGE ( 'NONE', *, *, #13039, .F. ) ;
#22692=CARTESIAN_POINT ( 'NONE',  ( -34.49999999999998579, -28.31857036507959791, 80.03062855292519373 ) ) ;
#22723=CARTESIAN_POINT ( 'NONE',  ( -42.49999999999999289, -21.76666049839542438, 84.29903810567665801 ) ) ;
#22743=FACE_OUTER_BOUND ( 'NONE', #2233, .T. ) ;
#22758=CARTESIAN_POINT ( 'NONE',  ( -42.49999999999999289, -39.95319397786859383, 75.20096189432314304 ) ) ;
#22762=CARTESIAN_POINT ( 'NONE',  ( -42.49999999999999289, -25.98076211353320986, 84.99999999999994316 ) ) ;
#22776=CYLINDRICAL_SURFACE ( 'NONE', #9582, 13.99999999999999822 ) ;
#22784=FACE_OUTER_BOUND ( 'NONE', #14450, .T. ) ;
#22830=EDGE_CURVE ( 'NONE', #793, #12715, #24860, .T. ) ;
#22902=EDGE_CURVE ( 'NONE', #29247, #32761, #34656, .T. ) ;
#22967=ORIENTED_EDGE ( 'NONE', *, *, #10637, .F. ) ;
#23005=ORIENTED_EDGE ( 'NONE', *, *, #28049, .T. ) ;
#23015=DIRECTION ( 'NONE',  ( -1.734723475976807094E-16, -0.4999999999999928946, -0.8660254037844427044 ) ) ;
#23018=ORIENTED_EDGE ( 'NONE', *, *, #19154, .F. ) ;
#23021=ORIENTED_EDGE ( 'NONE', *, *, #24985, .F. ) ;
#23051=DIRECTION ( 'NONE',  ( -1.734723475976806848E-16, -0.8660254037844350439, -0.5000000000000061062 ) ) ;
#23062=ADVANCED_FACE ( 'NONE', ( #20912 ), #31909, .F. ) ;
#23079=DIRECTION ( 'NONE',  ( 0.000000000000000000, -1.000000000000000000, 0.000000000000000000 ) ) ;
#23110=AXIS2_PLACEMENT_3D ( 'NONE', #1041, #34522, #23527 ) ;
#23148=ORIENTED_EDGE ( 'NONE', *, *, #230, .T. ) ;
#23172=CARTESIAN_POINT ( 'NONE',  ( -34.49999999999998579, -21.98076211353320630, 84.99999999999994316 ) ) ;
#23195=ORIENTED_EDGE ( 'NONE', *, *, #26677, .T. ) ;
#23208=ORIENTED_EDGE ( 'NONE', *, *, #35495, .F. ) ;
#23228=EDGE_CURVE ( 'NONE', #29583, #3694, #1798, .T. ) ;
#23282=CARTESIAN_POINT ( 'NONE',  ( -21.15833593587365513, -12.00833024919776371, 94.79903810567661537 ) ) ;
#23287=AXIS2_PLACEMENT_3D ( 'NONE', #9114, #25332, #6410 ) ;
#23296=VECTOR ( 'NONE', #28992, 1000.000000000000114 ) ;
#23301=CARTESIAN_POINT ( 'NONE',  ( -34.49999999999998579, -25.27980021920980036, 80.78589838486217900 ) ) ;
#23328=DIRECTION ( 'NONE',  ( 0.000000000000000000, 0.5000000000000092149, -0.8660254037844333785 ) ) ;
#23347=CARTESIAN_POINT ( 'NONE',  ( -34.49999999999998579, -14.60640646055094649, 76.70096189432339884 ) ) ;
#23360=DIRECTION ( 'NONE',  ( 0.000000000000000000, 1.000000000000000000, -1.067522139062650474E-15 ) ) ;
#23364=VECTOR ( 'NONE', #381, 1000.000000000000000 ) ;
#23382=ADVANCED_FACE ( 'NONE', ( #23396 ), #15091, .T. ) ;
#23396=FACE_OUTER_BOUND ( 'NONE', #30637, .T. ) ;
#23421=DIRECTION ( 'NONE',  ( 1.226634733346697831E-16, -0.2588190451025308425, 0.9659258262890655367 ) ) ;
#23423=AXIS2_PLACEMENT_3D ( 'NONE', #1578, #12372, #9843 ) ;
#23446=EDGE_CURVE ( 'NONE', #9169, #11290, #28370, .T. ) ;
#23448=EDGE_LOOP ( 'NONE', ( #29595, #19078, #7941, #13461 ) ) ;
#23459=DIRECTION ( 'NONE',  ( 0.000000000000000000, 1.000000000000000000, 0.000000000000000000 ) ) ;
#23461=FACE_OUTER_BOUND ( 'NONE', #33026, .T. ) ;
#23463=VECTOR ( 'NONE', #23015, 1000.000000000000227 ) ;
#23466=CARTESIAN_POINT ( 'NONE',  ( -34.49999999999998579, -14.67619866229190784, 76.74125644078590369 ) ) ;
#23468=LINE ( 'NONE', #6897, #20735 ) ;
#23499=VECTOR ( 'NONE', #29925, 1000.000000000000000 ) ;
#23527=DIRECTION ( 'NONE',  ( 0.000000000000000000, -1.000000000000000000, 0.000000000000000000 ) ) ;
#23548=DIRECTION ( 'NONE',  ( -1.734723475976807094E-16, 0.5000000000000092149, -0.8660254037844333785 ) ) ;
#23558=VECTOR ( 'NONE', #28374, 1000.000000000000114 ) ;
#23599=DIRECTION ( 'NONE',  ( -1.000000000000000000, -1.502314598737158292E-16, -8.673617379884052728E-17 ) ) ;
#23609=VECTOR ( 'NONE', #1058, 1000.000000000000000 ) ;
#23668=DIRECTION ( 'NONE',  ( 1.000000000000000000, 1.734723475976807094E-16, 0.000000000000000000 ) ) ;
#23698=VERTEX_POINT ( 'NONE', #30923 ) ;
#23703=CARTESIAN_POINT ( 'NONE',  ( -34.49999999999998579, -21.98076211353320630, 84.99999999999994316 ) ) ;
#23707=ORIENTED_EDGE ( 'NONE', *, *, #8348, .T. ) ;
#23795=ORIENTED_EDGE ( 'NONE', *, *, #26936, .T. ) ;
#23799=DIRECTION ( 'NONE',  ( 0.000000000000000000, -2.423959199780483078E-15, 1.000000000000000000 ) ) ;
#23808=CIRCLE ( 'NONE', #3099, 4.000000000000003553 ) ;
#23851=DIRECTION ( 'NONE',  ( -1.000000000000000000, -1.734723475976807094E-16, -0.000000000000000000 ) ) ;
#23856=DIRECTION ( 'NONE',  ( 0.000000000000000000, 1.000000000000000000, -1.067522139062650474E-15 ) ) ;
#23862=PLANE ( 'NONE',  #12470 ) ;
#23880=DIRECTION ( 'NONE',  ( 1.000000000000000000, 1.734723475976807094E-16, 0.000000000000000000 ) ) ;
#23914=ORIENTED_EDGE ( 'NONE', *, *, #24071, .F. ) ;
#23924=EDGE_LOOP ( 'NONE', ( #7565, #14236, #20787, #32293 ) ) ;
#23940=CARTESIAN_POINT ( 'NONE',  ( -21.15833593587365513, -8.980762113533204527, 86.49999999999994316 ) ) ;
#23941=ORIENTED_EDGE ( 'NONE', *, *, #33710, .F. ) ;
#23943=CARTESIAN_POINT ( 'NONE',  ( -34.49999999999998579, -25.98076211353322051, 84.99999999999992895 ) ) ;
#23971=VECTOR ( 'NONE', #17947, 1000.000000000000000 ) ;
#23978=AXIS2_PLACEMENT_3D ( 'NONE', #294, #11282, #22254 ) ;
#24022=PLANE ( 'NONE',  #370 ) ;
#24025=ORIENTED_EDGE ( 'NONE', *, *, #34831, .T. ) ;
#24034=EDGE_CURVE ( 'NONE', #25299, #32530, #1944, .T. ) ;
#24037=AXIS2_PLACEMENT_3D ( 'NONE', #1077, #34020, #19945 ) ;
#24046=EDGE_CURVE ( 'NONE', #19124, #26081, #23808, .T. ) ;
#24054=CYLINDRICAL_SURFACE ( 'NONE', #27985, 13.99999999999999822 ) ;
#24055=AXIS2_PLACEMENT_3D ( 'NONE', #15689, #12477, #13019 ) ;
#24071=EDGE_CURVE ( 'NONE', #32406, #17996, #32178, .T. ) ;
#24089=VECTOR ( 'NONE', #12326, 1000.000000000000000 ) ;
#24121=DIRECTION ( 'NONE',  ( 1.000000000000000000, 1.734723475976807094E-16, 0.000000000000000000 ) ) ;
#24142=CARTESIAN_POINT ( 'NONE',  ( -42.49999999999999289, -26.94801722181404102, 85.25380613764170334 ) ) ;
#24192=VERTEX_POINT ( 'NONE', #17146 ) ;
#24207=( GEOMETRIC_REPRESENTATION_CONTEXT ( 3 ) GLOBAL_UNCERTAINTY_ASSIGNED_CONTEXT ( ( #33720 ) ) GLOBAL_UNIT_ASSIGNED_CONTEXT ( ( #21507, #18645, #2641 ) ) REPRESENTATION_CONTEXT ( 'NONE', 'WORKASPACE' ) );
#24208=VECTOR ( 'NONE', #12095, 1000.000000000000000 ) ;
#24214=CARTESIAN_POINT ( 'NONE',  ( -34.49999999999998579, -20.32009476567218798, 72.19543654875879213 ) ) ;
#24272=EDGE_CURVE ( 'NONE', #32986, #34870, #31562, .T. ) ;
#24281=CARTESIAN_POINT ( 'NONE',  ( -21.15833593587365513, -42.98076211353323828, 83.49999999999991473 ) ) ;
#24296=EDGE_LOOP ( 'NONE', ( #4679, #34548, #10946, #4504 ) ) ;
#24318=EDGE_CURVE ( 'NONE', #16181, #26147, #31911, .T. ) ;
#24332=ORIENTED_EDGE ( 'NONE', *, *, #2752, .F. ) ;
#24376=LINE ( 'NONE', #21656, #34418 ) ;
#24396=LINE ( 'NONE', #26935, #5610 ) ;
#24408=LINE ( 'NONE', #10192, #4409 ) ;
#24418=DIRECTION ( 'NONE',  ( -1.734723475976807094E-16, 0.8660254037844444808, -0.4999999999999898415 ) ) ;
#24432=ADVANCED_FACE ( 'NONE', ( #34802 ), #10665, .F. ) ;
#24436=AXIS2_PLACEMENT_3D ( 'NONE', #33964, #8925, #30902 ) ;
#24482=VERTEX_POINT ( 'NONE', #13016 ) ;
#24490=EDGE_CURVE ( 'NONE', #9715, #6623, #20975, .T. ) ;
#24493=ORIENTED_EDGE ( 'NONE', *, *, #16267, .F. ) ;
#24494=ORIENTED_EDGE ( 'NONE', *, *, #24490, .T. ) ;
#24495=DIRECTION ( 'NONE',  ( 0.000000000000000000, -0.5000000000000032196, 0.8660254037844368202 ) ) ;
#24546=DIRECTION ( 'NONE',  ( 0.000000000000000000, -0.8660254037844392627, 0.4999999999999989453 ) ) ;
#24558=CARTESIAN_POINT ( 'NONE',  ( -34.49999999999998579, -31.64142946139395107, 72.19543654875866423 ) ) ;
#24565=CARTESIAN_POINT ( 'NONE',  ( -42.49999999999999289, -29.27980021920983944, 82.28589838486210795 ) ) ;
#24571=VECTOR ( 'NONE', #12704, 1000.000000000000227 ) ;
#24577=DIRECTION ( 'NONE',  ( -1.000000000000000000, 0.000000000000000000, 0.000000000000000000 ) ) ;
#24605=VECTOR ( 'NONE', #27560, 1000.000000000000227 ) ;
#24613=CARTESIAN_POINT ( 'NONE',  ( -21.15833593587365513, -8.980762113533204527, 86.49999999999994316 ) ) ;
#24656=EDGE_CURVE ( 'NONE', #26147, #4012, #11542, .T. ) ;
#24678=PLANE ( 'NONE',  #33811 ) ;
#24703=DIRECTION ( 'NONE',  ( -1.000000000000000000, -8.673617379884210501E-17, 1.502314598737149170E-16 ) ) ;
#24706=EDGE_CURVE ( 'NONE', #7199, #7407, #3101, .T. ) ;
#24722=DIRECTION ( 'NONE',  ( 0.000000000000000000, 0.8660254037844410391, -0.4999999999999958367 ) ) ;
#24736=CARTESIAN_POINT ( 'NONE',  ( -34.49999999999998579, -17.72201855431906736, 96.30456345124113682 ) ) ;
#24740=AXIS2_PLACEMENT_3D ( 'NONE', #4420, #4604, #9441 ) ;
#24768=CARTESIAN_POINT ( 'NONE',  ( -42.49999999999999289, -24.48076211353301801, 67.99999999999991473 ) ) ;
#24773=FILL_AREA_STYLE ('',( #19175 ) ) ;
#24786=LINE ( 'NONE', #2657, #11931 ) ;
#24796=DIRECTION ( 'NONE',  ( 0.000000000000000000, -0.5000000000000092149, 0.8660254037844333785 ) ) ;
#24805=EDGE_LOOP ( 'NONE', ( #4308, #20715, #20429, #28790 ) ) ;
#24819=LINE ( 'NONE', #8245, #6308 ) ;
#24860=CIRCLE ( 'NONE', #29467, 14.00000000000000000 ) ;
#24863=EDGE_LOOP ( 'NONE', ( #10503, #15893, #33673, #21240, #17710, #12083 ) ) ;
#24882=CARTESIAN_POINT ( 'NONE',  ( -42.49999999999999289, -25.98076211353320986, 84.99999999999994316 ) ) ;
#24943=ORIENTED_EDGE ( 'NONE', *, *, #32146, .T. ) ;
#24952=AXIS2_PLACEMENT_3D ( 'NONE', #7026, #17466, #4347 ) ;
#24968=FACE_OUTER_BOUND ( 'NONE', #35167, .T. ) ;
#24984=EDGE_CURVE ( 'NONE', #14069, #27933, #4340, .T. ) ;
#24985=EDGE_CURVE ( 'NONE', #34324, #10214, #29541, .T. ) ;
#24992=VECTOR ( 'NONE', #13261, 1000.000000000000114 ) ;
#25013=ORIENTED_EDGE ( 'NONE', *, *, #745, .T. ) ;
#25023=ORIENTED_EDGE ( 'NONE', *, *, #6869, .F. ) ;
#25050=CARTESIAN_POINT ( 'NONE',  ( -34.49999999999998579, -36.56745899286266166, 87.83669687932923864 ) ) ;
#25058=ORIENTED_EDGE ( 'NONE', *, *, #18312, .T. ) ;
#25079=ORIENTED_EDGE ( 'NONE', *, *, #26918, .T. ) ;
#25081=CARTESIAN_POINT ( 'NONE',  ( -34.50000000000001421, -27.48076211353330578, 101.9999999999999432 ) ) ;
#25091=VECTOR ( 'NONE', #23599, 1000.000000000000000 ) ;
#25103=LINE ( 'NONE', #9070, #33372 ) ;
#25147=CARTESIAN_POINT ( 'NONE',  ( -42.49999999999999289, -10.50833024919765180, 77.79903810567678590 ) ) ;
#25176=ORIENTED_EDGE ( 'NONE', *, *, #1582, .F. ) ;
#25177=VERTEX_POINT ( 'NONE', #27194 ) ;
#25227=PLANE ( 'NONE',  #5921 ) ;
#25247=CARTESIAN_POINT ( 'NONE',  ( -34.49999999999998579, -25.98076211353322051, 84.99999999999992895 ) ) ;
#25276=DIRECTION ( 'NONE',  ( 1.000000000000000000, 1.734723475976807094E-16, 0.000000000000000000 ) ) ;
#25279=AXIS2_PLACEMENT_3D ( 'NONE', #7545, #4862, #15803 ) ;
#25283=DIRECTION ( 'NONE',  ( -1.226634733346697831E-16, 0.7071067811865557884, -0.7071067811865392461 ) ) ;
#25299=VERTEX_POINT ( 'NONE', #3951 ) ;
#25314=EDGE_CURVE ( 'NONE', #29087, #34324, #25905, .T. ) ;
#25324=DIRECTION ( 'NONE',  ( 1.000000000000000000, 0.000000000000000000, 0.000000000000000000 ) ) ;
#25332=DIRECTION ( 'NONE',  ( -1.000000000000000000, -1.734723475976807094E-16, -0.000000000000000000 ) ) ;
#25333=DIRECTION ( 'NONE',  ( 0.000000000000000000, 0.9672551082808338307, -0.2538061376417690695 ) ) ;
#25336=ORIENTED_EDGE ( 'NONE', *, *, #5090, .F. ) ;
#25339=DIRECTION ( 'NONE',  ( -1.734723475976807094E-16, -0.4999999999999928946, -0.8660254037844427044 ) ) ;
#25385=ORIENTED_EDGE ( 'NONE', *, *, #24034, .F. ) ;
#25412=CARTESIAN_POINT ( 'NONE',  ( -34.49999999999998579, -28.31857036507959791, 80.03062855292519373 ) ) ;
#25437=EDGE_LOOP ( 'NONE', ( #26323, #20669, #33178, #31750 ) ) ;
#25444=ORIENTED_EDGE ( 'NONE', *, *, #33488, .F. ) ;
#25468=ORIENTED_EDGE ( 'NONE', *, *, #18898, .F. ) ;
#25479=EDGE_LOOP ( 'NONE', ( #34206, #32038, #30147, #6370 ) ) ;
#25480=LINE ( 'NONE', #22231, #21768 ) ;
#25498=AXIS2_PLACEMENT_3D ( 'NONE', #21926, #24121, #35284 ) ;
#25506=CARTESIAN_POINT ( 'NONE',  ( -21.15833593587365513, -25.27980021920989984, 89.21410161513770731 ) ) ;
#25511=CARTESIAN_POINT ( 'NONE',  ( -34.50000000000001421, -18.77980021920990694, 100.4724318643354053 ) ) ;
#25526=VECTOR ( 'NONE', #29486, 1000.000000000000227 ) ;
#25537=APPLICATION_CONTEXT ( 'automotive_design' ) ;
#25557=CARTESIAN_POINT ( 'NONE',  ( -42.49999999999999289, -28.69486372867102375, 88.29903810567654432 ) ) ;
#25655=ORIENTED_EDGE ( 'NONE', *, *, #5805, .F. ) ;
#25673=PLANE ( 'NONE',  #2555 ) ;
#25681=CARTESIAN_POINT ( 'NONE',  ( -42.49999999999999289, -21.76666049839546346, 85.70096189432329936 ) ) ;
#25731=ADVANCED_FACE ( 'NONE', ( #30194 ), #5531, .T. ) ;
#25788=EDGE_CURVE ( 'NONE', #11685, #34870, #32527, .T. ) ;
#25855=CIRCLE ( 'NONE', #29865, 14.00000000000000000 ) ;
#25899=CIRCLE ( 'NONE', #24740, 14.00000000000000000 ) ;
#25905=LINE ( 'NONE', #6802, #19858 ) ;
#25912=DIRECTION ( 'NONE',  ( -1.000000000000000000, -8.673617379884000959E-17, -1.502314598737161250E-16 ) ) ;
#25989=CARTESIAN_POINT ( 'NONE',  ( -34.49999999999998579, -30.19486372867095980, 84.29903810567654432 ) ) ;
#26001=EDGE_CURVE ( 'NONE', #21432, #4018, #15028, .T. ) ;
#26054=DIRECTION ( 'NONE',  ( 0.000000000000000000, 1.000000000000000000, -1.067522139062650474E-15 ) ) ;
#26058=DIRECTION ( 'NONE',  ( 0.000000000000000000, 0.5000000000000092149, -0.8660254037844333785 ) ) ;
#26067=FACE_OUTER_BOUND ( 'NONE', #5339, .T. ) ;
#26081=VERTEX_POINT ( 'NONE', #1723 ) ;
#26086=ORIENTED_EDGE ( 'NONE', *, *, #7055, .F. ) ;
#26113=CARTESIAN_POINT ( 'NONE',  ( -34.49999999999998579, -29.98076211353323473, 83.49999999999990052 ) ) ;
#26125=ORIENTED_EDGE ( 'NONE', *, *, #19446, .F. ) ;
#26136=EDGE_LOOP ( 'NONE', ( #20909, #31010, #34475, #29672 ) ) ;
#26137=VERTEX_POINT ( 'NONE', #33033 ) ;
#26147=VERTEX_POINT ( 'NONE', #2813 ) ;
#26161=AXIS2_PLACEMENT_3D ( 'NONE', #21621, #15686, #26704 ) ;
#26169=CARTESIAN_POINT ( 'NONE',  ( -34.50000000000001421, -35.77980021920998155, 98.97243186433534845 ) ) ;
#26176=DIRECTION ( 'NONE',  ( -1.000000000000000000, -0.000000000000000000, 0.000000000000000000 ) ) ;
#26217=DIRECTION ( 'NONE',  ( 0.000000000000000000, 0.4999999999999989453, 0.8660254037844392627 ) ) ;
#26241=DIRECTION ( 'NONE',  ( 1.000000000000000000, 1.734723475976807094E-16, 0.000000000000000000 ) ) ;
#26282=DIRECTION ( 'NONE',  ( 1.000000000000000000, 0.000000000000000000, 0.000000000000000000 ) ) ;
#26287=AXIS2_PLACEMENT_3D ( 'NONE', #25247, #17119, #14066 ) ;
#26292=VECTOR ( 'NONE', #25339, 1000.000000000000227 ) ;
#26294=CARTESIAN_POINT ( 'NONE',  ( -42.49999999999999289, -31.64142946139416424, 97.80456345124107997 ) ) ;
#26323=ORIENTED_EDGE ( 'NONE', *, *, #34999, .F. ) ;
#26357=DIRECTION ( 'NONE',  ( 1.000000000000000000, 1.734723475976807094E-16, 0.000000000000000000 ) ) ;
#26395=EDGE_LOOP ( 'NONE', ( #28468, #25023, #16736, #24332 ) ) ;
#26402=DIRECTION ( 'NONE',  ( -1.000000000000000000, 1.734723475976807094E-16, 0.000000000000000000 ) ) ;
#26413=CARTESIAN_POINT ( 'NONE',  ( -42.49999999999999289, -27.93100416606583991, 81.50764321173598148 ) ) ;
#26453=VECTOR ( 'NONE', #35055, 1000.000000000000000 ) ;
#26460=VERTEX_POINT ( 'NONE', #18370 ) ;
#26465=VECTOR ( 'NONE', #67, 1000.000000000000114 ) ;
#26507=EDGE_CURVE ( 'NONE', #31835, #21432, #18901, .T. ) ;
#26518=EDGE_LOOP ( 'NONE', ( #19811, #25013, #22349, #1722 ) ) ;
#26521=DIRECTION ( 'NONE',  ( 1.000000000000000000, 1.734723475976807094E-16, 0.000000000000000000 ) ) ;
#26549=CIRCLE ( 'NONE', #8117, 14.00000000000000000 ) ;
#26561=LINE ( 'NONE', #1897, #29345 ) ;
#26565=ORIENTED_EDGE ( 'NONE', *, *, #18274, .F. ) ;
#26573=LINE ( 'NONE', #34675, #2650 ) ;
#26585=CARTESIAN_POINT ( 'NONE',  ( -34.49999999999998579, -39.90017302060828541, 86.49999999999991473 ) ) ;
#26589=CARTESIAN_POINT ( 'NONE',  ( 0.000000000000000000, 0.000000000000000000, 0.000000000000000000 ) ) ;
#26677=EDGE_CURVE ( 'NONE', #33126, #5490, #3066, .T. ) ;
#26682=DIRECTION ( 'NONE',  ( 0.000000000000000000, 0.8660254037844350439, 0.5000000000000061062 ) ) ;
#26694=VERTEX_POINT ( 'NONE', #19430 ) ;
#26704=DIRECTION ( 'NONE',  ( 0.000000000000000000, 1.000000000000000000, 0.000000000000000000 ) ) ;
#26721=DIRECTION ( 'NONE',  ( 1.226634733346697831E-16, -0.7071067811865466846, -0.7071067811865483499 ) ) ;
#26727=LINE ( 'NONE', #27255, #33074 ) ;
#26755=FACE_OUTER_BOUND ( 'NONE', #10449, .T. ) ;
#26756=CARTESIAN_POINT ( 'NONE',  ( -34.49999999999998579, -25.98076211353322051, 84.99999999999992895 ) ) ;
#26769=SURFACE_STYLE_USAGE ( .BOTH. , #8365 ) ;
#26771=VERTEX_POINT ( 'NONE', #12216 ) ;
#26794=CARTESIAN_POINT ( 'NONE',  ( -34.49999999999998579, -24.48076211353304998, 71.08058909292489602 ) ) ;
#26803=VECTOR ( 'NONE', #969, 1000.000000000000000 ) ;
#26809=VECTOR ( 'NONE', #31436, 1000.000000000000114 ) ;
#26821=DIRECTION ( 'NONE',  ( 0.000000000000000000, 1.000000000000000000, 0.000000000000000000 ) ) ;
#26835=CARTESIAN_POINT ( 'NONE',  ( -42.49999999999999289, -35.77980021920998155, 98.97243186433534845 ) ) ;
#26886=VECTOR ( 'NONE', #952, 1000.000000000000000 ) ;
#26918=EDGE_CURVE ( 'NONE', #16800, #19176, #14901, .T. ) ;
#26932=DIRECTION ( 'NONE',  ( 0.000000000000000000, 1.000000000000000000, 0.000000000000000000 ) ) ;
#26935=CARTESIAN_POINT ( 'NONE',  ( -21.15833593587365513, -34.27980021920977549, 73.62564434701768334 ) ) ;
#26936=EDGE_CURVE ( 'NONE', #9715, #19677, #6984, .T. ) ;
#26968=ADVANCED_FACE ( 'NONE', ( #12754 ), #29322, .F. ) ;
#27057=DIRECTION ( 'NONE',  ( 0.000000000000000000, -9.406921877466749789E-15, 1.000000000000000000 ) ) ;
#27065=LINE ( 'NONE', #13732, #930 ) ;
#27075=ORIENTED_EDGE ( 'NONE', *, *, #26507, .F. ) ;
#27118=DIRECTION ( 'NONE',  ( 1.000000000000000000, 0.000000000000000000, 0.000000000000000000 ) ) ;
#27129=ORIENTED_EDGE ( 'NONE', *, *, #32174, .F. ) ;
#27140=DIRECTION ( 'NONE',  ( -1.000000000000000000, 0.000000000000000000, 0.000000000000000000 ) ) ;
#27153=ORIENTED_EDGE ( 'NONE', *, *, #1064, .F. ) ;
#27156=CARTESIAN_POINT ( 'NONE',  ( -42.49999999999999289, -33.18172400785640264, 69.52756813566438154 ) ) ;
#27165=VERTEX_POINT ( 'NONE', #2851 ) ;
#27194=CARTESIAN_POINT ( 'NONE',  ( -42.49999999999999289, -24.48076211353304288, 71.08058909292489602 ) ) ;
#27197=VERTEX_POINT ( 'NONE', #29855 ) ;
#27233=DIRECTION ( 'NONE',  ( -1.734723475976807094E-16, 9.406921877466749789E-15, -1.000000000000000000 ) ) ;
#27253=ORIENTED_EDGE ( 'NONE', *, *, #7274, .T. ) ;
#27255=CARTESIAN_POINT ( 'NONE',  ( -34.49999999999998579, -28.31857036507959791, 80.03062855292519373 ) ) ;
#27257=ORIENTED_EDGE ( 'NONE', *, *, #5727, .T. ) ;
#27272=ADVANCED_FACE ( 'NONE', ( #28741 ), #9294, .T. ) ;
#27283=CARTESIAN_POINT ( 'NONE',  ( -42.49999999999999289, -37.35511776651544125, 93.29903810567650169 ) ) ;
#27317=CARTESIAN_POINT ( 'NONE',  ( -34.49999999999998579, -12.06135120645816983, 86.49999999999994316 ) ) ;
#27321=LINE ( 'NONE', #30195, #22151 ) ;
#27342=ADVANCED_FACE ( 'NONE', ( #33420 ), #15036, .F. ) ;
#27356=ADVANCED_FACE ( 'NONE', ( #22784 ), #34142, .T. ) ;
#27379=CARTESIAN_POINT ( 'NONE',  ( -42.49999999999999289, -29.27980021920993536, 87.71410161513767889 ) ) ;
#27427=FACE_OUTER_BOUND ( 'NONE', #24296, .T. ) ;
#27434=ORIENTED_EDGE ( 'NONE', *, *, #18468, .T. ) ;
#27441=ORIENTED_EDGE ( 'NONE', *, *, #16474, .T. ) ;
#27448=VECTOR ( 'NONE', #7626, 1000.000000000000227 ) ;
#27450=CARTESIAN_POINT ( 'NONE',  ( -42.49999999999999289, -23.26666049839539951, 81.70096189432331357 ) ) ;
#27466=DIRECTION ( 'NONE',  ( 0.000000000000000000, -0.5000000000000001110, 0.8660254037844385966 ) ) ;
#27485=ORIENTED_EDGE ( 'NONE', *, *, #13039, .T. ) ;
#27520=LINE ( 'NONE', #27858, #27867 ) ;
#27521=VERTEX_POINT ( 'NONE', #31965 ) ;
#27527=EDGE_CURVE ( 'NONE', #8147, #9312, #1549, .T. ) ;
#27556=EDGE_CURVE ( 'NONE', #14069, #29093, #21587, .T. ) ;
#27560=DIRECTION ( 'NONE',  ( -1.226634733346697831E-16, -0.2588190451025240701, 0.9659258262890673130 ) ) ;
#27589=VECTOR ( 'NONE', #26282, 1000.000000000000000 ) ;
#27610=VECTOR ( 'NONE', #14004, 1000.000000000000000 ) ;
#27644=CARTESIAN_POINT ( 'NONE',  ( -42.49999999999999289, -20.32009476567239048, 97.80456345124112261 ) ) ;
#27655=AXIS2_PLACEMENT_3D ( 'NONE', #19570, #14184, #19737 ) ;
#27658=( NAMED_UNIT ( * ) PLANE_ANGLE_UNIT ( ) SI_UNIT ( $, .RADIAN. ) );
#27747=ORIENTED_EDGE ( 'NONE', *, *, #34331, .T. ) ;
#27749=ADVANCED_FACE ( 'NONE', ( #19847 ), #31212, .F. ) ;
#27800=ADVANCED_FACE ( 'NONE', ( #22743 ), #3153, .F. ) ;
#27817=DIRECTION ( 'NONE',  ( 0.000000000000000000, -1.000000000000000000, 0.000000000000000000 ) ) ;
#27843=DIRECTION ( 'NONE',  ( 1.000000000000000000, 0.000000000000000000, 0.000000000000000000 ) ) ;
#27846=LINE ( 'NONE', #13977, #18114 ) ;
#27857=LINE ( 'NONE', #305, #3300 ) ;
#27858=CARTESIAN_POINT ( 'NONE',  ( -42.49999999999999289, -25.01350700525237514, 84.74619386235816876 ) ) ;
#27859=VERTEX_POINT ( 'NONE', #30691 ) ;
#27867=VECTOR ( 'NONE', #2858, 1000.000000000000114 ) ;
#27890=ORIENTED_EDGE ( 'NONE', *, *, #7670, .F. ) ;
#27897=LINE ( 'NONE', #12040, #23463 ) ;
#27933=VERTEX_POINT ( 'NONE', #26169 ) ;
#27959=ORIENTED_EDGE ( 'NONE', *, *, #4952, .F. ) ;
#27977=VECTOR ( 'NONE', #24703, 1000.000000000000000 ) ;
#27979=ORIENTED_EDGE ( 'NONE', *, *, #20898, .F. ) ;
#27985=AXIS2_PLACEMENT_3D ( 'NONE', #20954, #1721, #31777 ) ;
#27987=DIRECTION ( 'NONE',  ( 0.000000000000000000, 0.9659258262890707547, -0.2588190451025116912 ) ) ;
#28049=EDGE_CURVE ( 'NONE', #10255, #25177, #16545, .T. ) ;
#28068=DIRECTION ( 'NONE',  ( 0.000000000000000000, -0.5000000000000001110, 0.8660254037844385966 ) ) ;
#28085=LINE ( 'NONE', #3597, #14587 ) ;
#28090=ORIENTED_EDGE ( 'NONE', *, *, #26001, .T. ) ;
#28109=CARTESIAN_POINT ( 'NONE',  ( -34.49999999999998579, -17.72201855431888973, 73.69543654875883476 ) ) ;
#28117=CARTESIAN_POINT ( 'NONE',  ( -42.49999999999999289, -39.90017302060827831, 86.49999999999991473 ) ) ;
#28158=LINE ( 'NONE', #31568, #26803 ) ;
#28172=ORIENTED_EDGE ( 'NONE', *, *, #6380, .F. ) ;
#28180=CARTESIAN_POINT ( 'NONE',  ( -34.50000000000001421, -8.980762113533204527, 86.49999999999994316 ) ) ;
#28188=AXIS2_PLACEMENT_3D ( 'NONE', #35490, #19252, #22136 ) ;
#28192=CARTESIAN_POINT ( 'NONE',  ( -34.49999999999998579, -27.48076211353328802, 98.91941090707497608 ) ) ;
#28202=CARTESIAN_POINT ( 'NONE',  ( -42.49999999999999289, -39.90017302060827831, 83.49999999999991473 ) ) ;
#28229=CARTESIAN_POINT ( 'NONE',  ( -34.49999999999998579, -14.67619866229204284, 93.25874355921412473 ) ) ;
#28233=CYLINDRICAL_SURFACE ( 'NONE', #27655, 13.99999999999999822 ) ;
#28244=DIRECTION ( 'NONE',  ( 1.000000000000000000, 1.734723475976807094E-16, 0.000000000000000000 ) ) ;
#28341=DIRECTION ( 'NONE',  ( 0.000000000000000000, 0.5000000000000031086, -0.8660254037844368202 ) ) ;
#28352=DIRECTION ( 'NONE',  ( 1.000000000000000000, 1.734723475976807094E-16, 0.000000000000000000 ) ) ;
#28368=CARTESIAN_POINT ( 'NONE',  ( -34.49999999999998579, -25.98076211353320986, 84.99999999999994316 ) ) ;
#28370=CIRCLE ( 'NONE', #25498, 14.00000000000000000 ) ;
#28374=DIRECTION ( 'NONE',  ( 1.226634733346697831E-16, 0.7071067811865507924, -0.7071067811865441310 ) ) ;
#28391=FACE_OUTER_BOUND ( 'NONE', #17695, .T. ) ;
#28401=EDGE_CURVE ( 'NONE', #17782, #8803, #29494, .T. ) ;
#28416=CARTESIAN_POINT ( 'NONE',  ( -42.49999999999999289, -29.98076211353323828, 86.49999999999990052 ) ) ;
#28417=DIRECTION ( 'NONE',  ( 1.000000000000000000, 0.000000000000000000, 0.000000000000000000 ) ) ;
#28419=ORIENTED_EDGE ( 'NONE', *, *, #13745, .T. ) ;
#28468=ORIENTED_EDGE ( 'NONE', *, *, #29600, .F. ) ;
#28510=DIRECTION ( 'NONE',  ( -1.000000000000000000, -0.000000000000000000, 0.000000000000000000 ) ) ;
#28552=DIRECTION ( 'NONE',  ( -1.734723475976807094E-16, 1.000000000000000000, -1.067522139062650474E-15 ) ) ;
#28560=DIRECTION ( 'NONE',  ( 0.000000000000000000, -0.8660254037844392627, 0.4999999999999989453 ) ) ;
#28578=PRODUCT_CONTEXT ( 'NONE', #7346, 'mechanical' ) ;
#28616=ADVANCED_FACE ( 'NONE', ( #5533 ), #19707, .F. ) ;
#28630=AXIS2_PLACEMENT_3D ( 'NONE', #3734, #14687, #26054 ) ;
#28640=ADVANCED_FACE ( 'NONE', ( #8392, #30381 ), #3019, .F. ) ;
#28653=AXIS2_PLACEMENT_3D ( 'NONE', #659, #3559, #30917 ) ;
#28708=ORIENTED_EDGE ( 'NONE', *, *, #3953, .T. ) ;
#28720=CARTESIAN_POINT ( 'NONE',  ( -34.49999999999998579, -28.31857036507959791, 80.03062855292519373 ) ) ;
#28741=FACE_OUTER_BOUND ( 'NONE', #34323, .T. ) ;
#28748=VERTEX_POINT ( 'NONE', #28202 ) ;
#28777=ORIENTED_EDGE ( 'NONE', *, *, #30419, .T. ) ;
#28790=ORIENTED_EDGE ( 'NONE', *, *, #21844, .F. ) ;
#28824=VERTEX_POINT ( 'NONE', #3375 ) ;
#28840=CARTESIAN_POINT ( 'NONE',  ( -34.49999999999998579, -34.23950567274729195, 73.69543654875865002 ) ) ;
#28863=CARTESIAN_POINT ( 'NONE',  ( -42.49999999999999289, -31.64142946139395107, 72.19543654875866423 ) ) ;
#28907=ADVANCED_FACE ( 'NONE', ( #26755, #35215 ), #21150, .T. ) ;
#28953=VECTOR ( 'NONE', #6089, 1000.000000000000000 ) ;
#28992=DIRECTION ( 'NONE',  ( -1.226634733346697831E-16, -0.9659258262890664248, -0.2588190451025275673 ) ) ;
#29024=ORIENTED_EDGE ( 'NONE', *, *, #16723, .F. ) ;
#29087=VERTEX_POINT ( 'NONE', #27283 ) ;
#29093=VERTEX_POINT ( 'NONE', #5673 ) ;
#29124=COLOUR_RGB ( '', 0.40784314, 0.44705882, 0.49803922) ;
#29141=ORIENTED_EDGE ( 'NONE', *, *, #23228, .F. ) ;
#29155=ADVANCED_FACE ( 'NONE', ( #12301 ), #14282, .T. ) ;
#29214=ORIENTED_EDGE ( 'NONE', *, *, #9420, .F. ) ;
#29228=CARTESIAN_POINT ( 'NONE',  ( -21.15833593587365513, -27.48076211353314591, 80.99999999999987210 ) ) ;
#29247=VERTEX_POINT ( 'NONE', #19845 ) ;
#29320=ADVANCED_FACE ( 'NONE', ( #10640 ), #19083, .T. ) ;
#29322=CYLINDRICAL_SURFACE ( 'NONE', #12946, 4.000000000000003553 ) ;
#29345=VECTOR ( 'NONE', #6923, 1000.000000000000000 ) ;
#29346=PLANE ( 'NONE',  #6903 ) ;
#29365=DIRECTION ( 'NONE',  ( -1.734723475976807094E-16, 0.4999999999999989453, 0.8660254037844392627 ) ) ;
#29429=CARTESIAN_POINT ( 'NONE',  ( -42.49999999999999289, -23.26666049839546702, 88.29903810567660116 ) ) ;
#29467=AXIS2_PLACEMENT_3D ( 'NONE', #17148, #25276, #8875 ) ;
#29475=EDGE_LOOP ( 'NONE', ( #34503, #6418, #2956, #12661 ) ) ;
#29486=DIRECTION ( 'NONE',  ( 1.226634733346697831E-16, 0.2588190451025240701, -0.9659258262890673130 ) ) ;
#29489=FACE_OUTER_BOUND ( 'NONE', #23924, .T. ) ;
#29494=LINE ( 'NONE', #16131, #11851 ) ;
#29515=ADVANCED_FACE ( 'NONE', ( #19765 ), #24678, .F. ) ;
#29525=CARTESIAN_POINT ( 'NONE',  ( -34.49999999999998579, -25.98076211353322051, 84.99999999999992895 ) ) ;
#29535=AXIS2_PLACEMENT_3D ( 'NONE', #15168, #11962, #26176 ) ;
#29541=LINE ( 'NONE', #7018, #23296 ) ;
#29545=ORIENTED_EDGE ( 'NONE', *, *, #10425, .F. ) ;
#29558=AXIS2_PLACEMENT_3D ( 'NONE', #21248, #17251, #33470 ) ;
#29583=VERTEX_POINT ( 'NONE', #882 ) ;
#29595=ORIENTED_EDGE ( 'NONE', *, *, #24034, .T. ) ;
#29600=EDGE_CURVE ( 'NONE', #7845, #17749, #6637, .T. ) ;
#29616=VECTOR ( 'NONE', #27233, 1000.000000000000000 ) ;
#29627=CARTESIAN_POINT ( 'NONE',  ( -42.49999999999999289, -27.48076211353329157, 98.91941090707497608 ) ) ;
#29672=ORIENTED_EDGE ( 'NONE', *, *, #34184, .F. ) ;
#29677=ADVANCED_FACE ( 'NONE', ( #12045 ), #9703, .T. ) ;
#29682=DIRECTION ( 'NONE',  ( 0.000000000000000000, -1.000000000000000000, -2.423959199780483078E-15 ) ) ;
#29692=EDGE_LOOP ( 'NONE', ( #19685, #13184, #28172, #4324 ) ) ;
#29695=AXIS2_PLACEMENT_3D ( 'NONE', #35467, #16170, #32932 ) ;
#29720=AXIS2_PLACEMENT_3D ( 'NONE', #7860, #13628, #11279 ) ;
#29776=FACE_OUTER_BOUND ( 'NONE', #21206, .T. ) ;
#29779=ORIENTED_EDGE ( 'NONE', *, *, #33690, .F. ) ;
#29805=LINE ( 'NONE', #13411, #34960 ) ;
#29841=CIRCLE ( 'NONE', #19463, 4.000000000000003553 ) ;
#29855=CARTESIAN_POINT ( 'NONE',  ( -42.49999999999999289, -14.67619866229190784, 76.74125644078590369 ) ) ;
#29865=AXIS2_PLACEMENT_3D ( 'NONE', #12285, #26521, #31719 ) ;
#29875=FACE_OUTER_BOUND ( 'NONE', #10907, .T. ) ;
#29892=ORIENTED_EDGE ( 'NONE', *, *, #22271, .T. ) ;
#29925=DIRECTION ( 'NONE',  ( -1.000000000000000000, -0.000000000000000000, 0.000000000000000000 ) ) ;
#29927=ADVANCED_FACE ( 'NONE', ( #32377 ), #7698, .T. ) ;
#29988=VECTOR ( 'NONE', #35418, 1000.000000000000000 ) ;
#29997=DIRECTION ( 'NONE',  ( 1.000000000000000000, 0.000000000000000000, 0.000000000000000000 ) ) ;
#30058=CARTESIAN_POINT ( 'NONE',  ( -21.15833593587365513, -21.76666049839546346, 85.70096189432329936 ) ) ;
#30075=CARTESIAN_POINT ( 'NONE',  ( -34.49999999999998579, -15.39406523420381490, 87.83669687932935233 ) ) ;
#30109=ORIENTED_EDGE ( 'NONE', *, *, #19236, .F. ) ;
#30137=VECTOR ( 'NONE', #23856, 1000.000000000000000 ) ;
#30147=ORIENTED_EDGE ( 'NONE', *, *, #2752, .T. ) ;
#30167=CARTESIAN_POINT ( 'NONE',  ( -21.15833593587365513, -31.68172400785665488, 97.87435565298206086 ) ) ;
#30177=CARTESIAN_POINT ( 'NONE',  ( -21.15833593587365513, -39.98076211353324538, 86.49999999999991473 ) ) ;
#30194=FACE_OUTER_BOUND ( 'NONE', #6865, .T. ) ;
#30195=CARTESIAN_POINT ( 'NONE',  ( -34.49999999999998579, -28.69486372867102020, 88.29903810567654432 ) ) ;
#30198=ORIENTED_EDGE ( 'NONE', *, *, #22659, .T. ) ;
#30239=DIRECTION ( 'NONE',  ( 0.000000000000000000, -1.000000000000000000, 0.000000000000000000 ) ) ;
#30250=ORIENTED_EDGE ( 'NONE', *, *, #7135, .F. ) ;
#30265=EDGE_LOOP ( 'NONE', ( #11210, #4680, #9895, #3563 ) ) ;
#30309=VECTOR ( 'NONE', #9814, 1000.000000000000114 ) ;
#30324=VECTOR ( 'NONE', #17578, 1000.000000000000000 ) ;
#30336=DIRECTION ( 'NONE',  ( -1.000000000000000000, 0.000000000000000000, 0.000000000000000000 ) ) ;
#30347=ORIENTED_EDGE ( 'NONE', *, *, #21810, .T. ) ;
#30348=( LENGTH_UNIT ( ) NAMED_UNIT ( * ) SI_UNIT ( .MILLI., .METRE. ) );
#30378=VECTOR ( 'NONE', #3482, 1000.000000000000000 ) ;
#30381=FACE_BOUND ( 'NONE', #750, .T. ) ;
#30419=EDGE_CURVE ( 'NONE', #11413, #14117, #26727, .T. ) ;
#30424=ORIENTED_EDGE ( 'NONE', *, *, #19446, .T. ) ;
#30430=ORIENTED_EDGE ( 'NONE', *, *, #19334, .F. ) ;
#30431=VECTOR ( 'NONE', #4774, 1000.000000000000000 ) ;
#30439=VERTEX_POINT ( 'NONE', #14257 ) ;
#30517=EDGE_CURVE ( 'NONE', #22358, #2456, #22181, .T. ) ;
#30525=EDGE_LOOP ( 'NONE', ( #18501, #33657, #21176, #10592 ) ) ;
#30544=DIRECTION ( 'NONE',  ( 0.000000000000000000, -0.4999999999999958367, -0.8660254037844410391 ) ) ;
#30586=DIRECTION ( 'NONE',  ( -1.000000000000000000, -1.734723475976807094E-16, -0.000000000000000000 ) ) ;
#30618=AXIS2_PLACEMENT_3D ( 'NONE', #19780, #11364, #22671 ) ;
#30631=EDGE_CURVE ( 'NONE', #6172, #26694, #34609, .T. ) ;
#30635=VECTOR ( 'NONE', #12775, 1000.000000000000000 ) ;
#30637=EDGE_LOOP ( 'NONE', ( #18247, #35483, #34105, #27890 ) ) ;
#30647=CARTESIAN_POINT ( 'NONE',  ( -42.49999999999999289, -14.60640646055094649, 76.70096189432339884 ) ) ;
#30686=DIRECTION ( 'NONE',  ( 0.000000000000000000, -9.406921877466749789E-15, 1.000000000000000000 ) ) ;
#30691=CARTESIAN_POINT ( 'NONE',  ( -42.49999999999999289, -33.18172400785640264, 69.52756813566438154 ) ) ;
#30693=VECTOR ( 'NONE', #34897, 1000.000000000000114 ) ;
#30698=ORIENTED_EDGE ( 'NONE', *, *, #7135, .T. ) ;
#30700=VERTEX_POINT ( 'NONE', #28840 ) ;
#30771=DIRECTION ( 'NONE',  ( 0.000000000000000000, -0.8660254037844410391, 0.4999999999999958367 ) ) ;
#30788=EDGE_CURVE ( 'NONE', #17135, #19278, #15312, .T. ) ;
#30817=LINE ( 'NONE', #11037, #2722 ) ;
#30840=LINE ( 'NONE', #22723, #26886 ) ;
#30847=AXIS2_PLACEMENT_3D ( 'NONE', #19545, #25333, #33593 ) ;
#30896=DIRECTION ( 'NONE',  ( 1.226634733346697831E-16, -0.9659258262890646485, -0.2588190451025342842 ) ) ;
#30902=DIRECTION ( 'NONE',  ( -1.000000000000000000, -0.000000000000000000, 0.000000000000000000 ) ) ;
#30917=DIRECTION ( 'NONE',  ( 0.000000000000000000, 1.000000000000000000, 0.000000000000000000 ) ) ;
#30923=CARTESIAN_POINT ( 'NONE',  ( -34.49999999999998579, -14.67619866229203929, 93.25874355921412473 ) ) ;
#30958=ORIENTED_EDGE ( 'NONE', *, *, #14757, .T. ) ;
#30966=CARTESIAN_POINT ( 'NONE',  ( -42.49999999999999289, -38.85511776651532756, 79.29903810567645905 ) ) ;
#30977=LINE ( 'NONE', #28109, #27977 ) ;
#31010=ORIENTED_EDGE ( 'NONE', *, *, #5774, .F. ) ;
#31011=PRODUCT_DEFINITION_CONTEXT ( 'detailed design', #25537, 'design' ) ;
#31031=DIRECTION ( 'NONE',  ( 0.000000000000000000, 0.4999999999999989453, 0.8660254037844392627 ) ) ;
#31089=EDGE_CURVE ( 'NONE', #12715, #1256, #8635, .T. ) ;
#31100=VERTEX_POINT ( 'NONE', #11869 ) ;
#31125=CARTESIAN_POINT ( 'NONE',  ( -34.49999999999998579, -17.72201855431907447, 96.30456345124113682 ) ) ;
#31136=ORIENTED_EDGE ( 'NONE', *, *, #11021, .F. ) ;
#31182=ORIENTED_EDGE ( 'NONE', *, *, #4723, .F. ) ;
#31198=CARTESIAN_POINT ( 'NONE',  ( -34.49999999999998579, -25.98076211353322051, 84.99999999999992895 ) ) ;
#31210=EDGE_CURVE ( 'NONE', #24482, #2498, #34026, .T. ) ;
#31211=VECTOR ( 'NONE', #29997, 1000.000000000000000 ) ;
#31212=CYLINDRICAL_SURFACE ( 'NONE', #31928, 4.000000000000003553 ) ;
#31219=CARTESIAN_POINT ( 'NONE',  ( -21.15833593587365513, -29.27980021920993536, 87.71410161513767889 ) ) ;
#31231=CARTESIAN_POINT ( 'NONE',  ( -42.49999999999999289, -25.98076211353322051, 84.99999999999992895 ) ) ;
#31276=LINE ( 'NONE', #4468, #17938 ) ;
#31395=DIRECTION ( 'NONE',  ( 0.000000000000000000, -0.8660254037844368202, -0.5000000000000031086 ) ) ;
#31419=DIRECTION ( 'NONE',  ( 0.000000000000000000, 0.8660254037844350439, 0.5000000000000061062 ) ) ;
#31420=ORIENTED_EDGE ( 'NONE', *, *, #34295, .F. ) ;
#31436=DIRECTION ( 'NONE',  ( 0.000000000000000000, -0.8660254037844410391, 0.4999999999999958367 ) ) ;
#31440=CARTESIAN_POINT ( 'NONE',  ( -42.49999999999999289, -25.27980021920979326, 80.78589838486217900 ) ) ;
#31551=VECTOR ( 'NONE', #7660, 1000.000000000000000 ) ;
#31562=LINE ( 'NONE', #14622, #17507 ) ;
#31568=CARTESIAN_POINT ( 'NONE',  ( -34.49999999999998579, -23.26666049839540307, 81.70096189432331357 ) ) ;
#31578=FACE_OUTER_BOUND ( 'NONE', #19205, .T. ) ;
#31595=VERTEX_POINT ( 'NONE', #20799 ) ;
#31600=DIRECTION ( 'NONE',  ( -1.734723475976807094E-16, 0.4999999999999989453, 0.8660254037844392627 ) ) ;
#31614=DIRECTION ( 'NONE',  ( -1.000000000000000000, 1.502314598737164455E-16, -8.673617379883947958E-17 ) ) ;
#31637=LINE ( 'NONE', #15237, #23971 ) ;
#31653=ORIENTED_EDGE ( 'NONE', *, *, #34331, .F. ) ;
#31668=CARTESIAN_POINT ( 'NONE',  ( -42.49999999999999289, -34.23950567274729195, 73.69543654875863581 ) ) ;
#31682=CARTESIAN_POINT ( 'NONE',  ( -34.49999999999998579, -34.23950567274729195, 73.69543654875863581 ) ) ;
#31719=DIRECTION ( 'NONE',  ( 0.000000000000000000, 1.000000000000000000, 0.000000000000000000 ) ) ;
#31731=EDGE_CURVE ( 'NONE', #2578, #31595, #17754, .T. ) ;
#31750=ORIENTED_EDGE ( 'NONE', *, *, #4723, .T. ) ;
#31758=CARTESIAN_POINT ( 'NONE',  ( -42.49999999999999289, -25.98076211353322051, 84.99999999999992895 ) ) ;
#31770=LINE ( 'NONE', #24214, #21478 ) ;
#31777=DIRECTION ( 'NONE',  ( 0.000000000000000000, -1.000000000000000000, 0.000000000000000000 ) ) ;
#31790=VECTOR ( 'NONE', #15185, 1000.000000000000000 ) ;
#31806=DIRECTION ( 'NONE',  ( -1.226634733346697831E-16, -0.9659258262890698665, 0.2588190451025151884 ) ) ;
#31835=VERTEX_POINT ( 'NONE', #26413 ) ;
#31842=CARTESIAN_POINT ( 'NONE',  ( -34.49999999999998579, -13.17619866229195047, 79.33933265213923391 ) ) ;
#31902=ADVANCED_FACE ( 'NONE', ( #2303 ), #31986, .F. ) ;
#31909=PLANE ( 'NONE',  #13956 ) ;
#31911=CIRCLE ( 'NONE', #15215, 14.00000000000000000 ) ;
#31916=DIRECTION ( 'NONE',  ( 0.000000000000000000, 1.000000000000000000, 0.000000000000000000 ) ) ;
#31928=AXIS2_PLACEMENT_3D ( 'NONE', #8885, #33556, #27817 ) ;
#31959=DIRECTION ( 'NONE',  ( 1.000000000000000000, 0.000000000000000000, -0.000000000000000000 ) ) ;
#31964=MECHANICAL_DESIGN_GEOMETRIC_PRESENTATION_REPRESENTATION('',(#6670),#10120);
#31965=CARTESIAN_POINT ( 'NONE',  ( -42.49999999999999289, -21.98076211353320630, 84.99999999999994316 ) ) ;
#31968=ORIENTED_EDGE ( 'NONE', *, *, #13487, .T. ) ;
#31986=PLANE ( 'NONE',  #3600 ) ;
#31989=CIRCLE ( 'NONE', #6129, 14.00000000000000000 ) ;
#32038=ORIENTED_EDGE ( 'NONE', *, *, #9326, .T. ) ;
#32146=EDGE_CURVE ( 'NONE', #25177, #34234, #19652, .T. ) ;
#32174=EDGE_CURVE ( 'NONE', #24192, #32530, #14473, .T. ) ;
#32178=LINE ( 'NONE', #12377, #25526 ) ;
#32214=CARTESIAN_POINT ( 'NONE',  ( -21.15833593587365513, -12.00833024919776371, 94.79903810567661537 ) ) ;
#32293=ORIENTED_EDGE ( 'NONE', *, *, #18468, .F. ) ;
#32318=DIRECTION ( 'NONE',  ( 1.000000000000000000, 1.734723475976807094E-16, 0.000000000000000000 ) ) ;
#32328=CARTESIAN_POINT ( 'NONE',  ( -42.49999999999999289, -13.17619866229195047, 79.33933265213923391 ) ) ;
#32377=FACE_OUTER_BOUND ( 'NONE', #26518, .T. ) ;
#32405=CARTESIAN_POINT ( 'NONE',  ( -42.49999999999999289, -24.48076211353301801, 67.99999999999991473 ) ) ;
#32406=VERTEX_POINT ( 'NONE', #18429 ) ;
#32435=ORIENTED_EDGE ( 'NONE', *, *, #18898, .T. ) ;
#32457=EDGE_CURVE ( 'NONE', #3694, #2456, #13755, .T. ) ;
#32466=ORIENTED_EDGE ( 'NONE', *, *, #1133, .T. ) ;
#32484=ORIENTED_EDGE ( 'NONE', *, *, #3742, .F. ) ;
#32527=LINE ( 'NONE', #25681, #21619 ) ;
#32530=VERTEX_POINT ( 'NONE', #30966 ) ;
#32573=CARTESIAN_POINT ( 'NONE',  ( -21.15833593587365513, -22.68172400785649501, 82.28589838486220742 ) ) ;
#32587=ORIENTED_EDGE ( 'NONE', *, *, #27527, .F. ) ;
#32636=EDGE_LOOP ( 'NONE', ( #1623, #12756, #27434, #25444 ) ) ;
#32677=CARTESIAN_POINT ( 'NONE',  ( -34.49999999999998579, -27.48076211353304998, 71.08058909292485339 ) ) ;
#32679=DIRECTION ( 'NONE',  ( -1.000000000000000000, 6.056754644426116516E-31, -1.734723475976807094E-16 ) ) ;
#32698=VECTOR ( 'NONE', #3553, 1000.000000000000000 ) ;
#32718=DIRECTION ( 'NONE',  ( 0.000000000000000000, 0.8660254037844333785, 0.5000000000000092149 ) ) ;
#32730=ORIENTED_EDGE ( 'NONE', *, *, #34096, .T. ) ;
#32748=DIRECTION ( 'NONE',  ( 1.226634733346697831E-16, 0.7071067811865466846, 0.7071067811865483499 ) ) ;
#32753=DIRECTION ( 'NONE',  ( 0.000000000000000000, 0.8660254037844333785, 0.5000000000000092149 ) ) ;
#32761=VERTEX_POINT ( 'NONE', #31668 ) ;
#32762=EDGE_CURVE ( 'NONE', #5490, #20834, #7003, .T. ) ;
#32777=ORIENTED_EDGE ( 'NONE', *, *, #8553, .F. ) ;
#32793=ADVANCED_FACE ( 'NONE', ( #1084 ), #12055, .F. ) ;
#32820=CYLINDRICAL_SURFACE ( 'NONE', #26287, 13.99999999999999822 ) ;
#32825=ORIENTED_EDGE ( 'NONE', *, *, #22830, .F. ) ;
#32827=ADVANCED_FACE ( 'NONE', ( #29875 ), #29346, .F. ) ;
#32907=DIRECTION ( 'NONE',  ( -1.000000000000000000, -1.502314598737170371E-16, 8.673617379883843187E-17 ) ) ;
#32930=FACE_OUTER_BOUND ( 'NONE', #13831, .T. ) ;
#32932=DIRECTION ( 'NONE',  ( 0.000000000000000000, 1.000000000000000000, 0.000000000000000000 ) ) ;
#32933=FACE_OUTER_BOUND ( 'NONE', #18222, .T. ) ;
#32937=CARTESIAN_POINT ( 'NONE',  ( -42.49999999999999289, -25.98076211353322051, 84.99999999999992895 ) ) ;
#32940=VECTOR ( 'NONE', #21229, 1000.000000000000000 ) ;
#32954=EDGE_CURVE ( 'NONE', #24482, #8147, #13799, .T. ) ;
#32966=VECTOR ( 'NONE', #4039, 1000.000000000000114 ) ;
#32986=VERTEX_POINT ( 'NONE', #19732 ) ;
#33001=ORIENTED_EDGE ( 'NONE', *, *, #31089, .F. ) ;
#33002=EDGE_CURVE ( 'NONE', #29093, #17785, #24819, .T. ) ;
#33011=DIRECTION ( 'NONE',  ( -1.734723475976807094E-16, 9.406921877466749789E-15, -1.000000000000000000 ) ) ;
#33017=VECTOR ( 'NONE', #12792, 1000.000000000000000 ) ;
#33026=EDGE_LOOP ( 'NONE', ( #20878, #18587, #830, #17572 ) ) ;
#33028=CARTESIAN_POINT ( 'NONE',  ( -34.49999999999998579, -23.26666049839546702, 88.29903810567660116 ) ) ;
#33033=CARTESIAN_POINT ( 'NONE',  ( -34.49999999999998579, -11.98076211353319742, 83.49999999999992895 ) ) ;
#33063=PLANE ( 'NONE',  #8752 ) ;
#33074=VECTOR ( 'NONE', #35018, 1000.000000000000114 ) ;
#33099=EDGE_LOOP ( 'NONE', ( #23021, #4153, #11872, #19320 ) ) ;
#33112=EDGE_CURVE ( 'NONE', #12635, #1256, #18640, .T. ) ;
#33126=VERTEX_POINT ( 'NONE', #22050 ) ;
#33128=LINE ( 'NONE', #30075, #24605 ) ;
#33133=CARTESIAN_POINT ( 'NONE',  ( -21.15833593587365513, -10.50833024919764469, 77.79903810567677169 ) ) ;
#33167=VECTOR ( 'NONE', #8575, 1000.000000000000114 ) ;
#33175=VECTOR ( 'NONE', #10677, 1000.000000000000000 ) ;
#33178=ORIENTED_EDGE ( 'NONE', *, *, #8871, .T. ) ;
#33207=VECTOR ( 'NONE', #24495, 999.9999999999998863 ) ;
#33239=CARTESIAN_POINT ( 'NONE',  ( -34.49999999999998579, -38.78532556477446036, 90.66066734786069503 ) ) ;
#33243=EDGE_CURVE ( 'NONE', #2456, #1876, #16100, .T. ) ;
#33257=LINE ( 'NONE', #298, #33167 ) ;
#33262=LINE ( 'NONE', #8579, #26292 ) ;
#33279=EDGE_LOOP ( 'NONE', ( #7082, #820, #33950, #19772 ) ) ;
#33359=ORIENTED_EDGE ( 'NONE', *, *, #22086, .F. ) ;
#33372=VECTOR ( 'NONE', #25283, 1000.000000000000000 ) ;
#33381=CARTESIAN_POINT ( 'NONE',  ( -21.15833593587365513, -39.95319397786859383, 75.20096189432314304 ) ) ;
#33391=( LENGTH_UNIT ( ) NAMED_UNIT ( * ) SI_UNIT ( .MILLI., .METRE. ) );
#33392=ORIENTED_EDGE ( 'NONE', *, *, #31731, .T. ) ;
#33420=FACE_OUTER_BOUND ( 'NONE', #33099, .T. ) ;
#33427=DIRECTION ( 'NONE',  ( 0.000000000000000000, 0.7071067811865483499, -0.7071067811865466846 ) ) ;
#33429=ORIENTED_EDGE ( 'NONE', *, *, #8348, .F. ) ;
#33430=EDGE_CURVE ( 'NONE', #7962, #17785, #4496, .T. ) ;
#33432=EDGE_CURVE ( 'NONE', #15848, #34028, #33128, .T. ) ;
#33449=CARTESIAN_POINT ( 'NONE',  ( -42.49999999999999289, -11.98076211353319742, 83.49999999999992895 ) ) ;
#33470=DIRECTION ( 'NONE',  ( 0.000000000000000000, 1.000000000000000000, 0.000000000000000000 ) ) ;
#33488=EDGE_CURVE ( 'NONE', #7962, #22358, #5243, .T. ) ;
#33516=CARTESIAN_POINT ( 'NONE',  ( -21.15833593587365513, -28.69486372867102375, 88.29903810567654432 ) ) ;
#33536=DIRECTION ( 'NONE',  ( 0.000000000000000000, 0.8660254037844428154, -0.4999999999999929501 ) ) ;
#33556=DIRECTION ( 'NONE',  ( -1.000000000000000000, -1.734723475976807094E-16, -0.000000000000000000 ) ) ;
#33584=LINE ( 'NONE', #25147, #3182 ) ;
#33593=DIRECTION ( 'NONE',  ( 0.000000000000000000, 0.2538061376417690140, 0.9672551082808337197 ) ) ;
#33596=ORIENTED_EDGE ( 'NONE', *, *, #8871, .F. ) ;
#33657=ORIENTED_EDGE ( 'NONE', *, *, #7055, .T. ) ;
#33663=FACE_OUTER_BOUND ( 'NONE', #26136, .T. ) ;
#33673=ORIENTED_EDGE ( 'NONE', *, *, #30419, .F. ) ;
#33690=EDGE_CURVE ( 'NONE', #17785, #29087, #3070, .T. ) ;
#33710=EDGE_CURVE ( 'NONE', #16181, #532, #27897, .T. ) ;
#33720=UNCERTAINTY_MEASURE_WITH_UNIT (LENGTH_MEASURE( 1.000000000000000082E-05 ), #21507, 'distance_accuracy_value', 'NONE');
#33766=DIRECTION ( 'NONE',  ( 0.000000000000000000, 1.000000000000000000, 0.000000000000000000 ) ) ;
#33811=AXIS2_PLACEMENT_3D ( 'NONE', #33133, #8276, #22137 ) ;
#33898=CYLINDRICAL_SURFACE ( 'NONE', #4092, 13.99999999999999822 ) ;
#33909=ORIENTED_EDGE ( 'NONE', *, *, #22830, .T. ) ;
#33926=DIRECTION ( 'NONE',  ( -1.000000000000000000, -1.734723475976807094E-16, -0.000000000000000000 ) ) ;
#33933=EDGE_LOOP ( 'NONE', ( #29141, #35258, #28419, #15259 ) ) ;
#33937=EDGE_CURVE ( 'NONE', #6623, #27197, #2857, .T. ) ;
#33950=ORIENTED_EDGE ( 'NONE', *, *, #1665, .F. ) ;
#33964=CARTESIAN_POINT ( 'NONE',  ( -21.15833593587365513, -41.45319397786874305, 92.20096189432315725 ) ) ;
#33986=EDGE_LOOP ( 'NONE', ( #11359, #16438, #27153, #6832 ) ) ;
#34020=DIRECTION ( 'NONE',  ( -1.000000000000000000, -1.734723475976807094E-16, -0.000000000000000000 ) ) ;
#34026=LINE ( 'NONE', #31842, #10997 ) ;
#34028=VERTEX_POINT ( 'NONE', #25511 ) ;
#34042=CARTESIAN_POINT ( 'NONE',  ( -34.49999999999998579, -21.98076211353320630, 86.49999999999995737 ) ) ;
#34087=DIRECTION ( 'NONE',  ( 0.000000000000000000, -1.000000000000000000, 1.067522139062650474E-15 ) ) ;
#34094=CARTESIAN_POINT ( 'NONE',  ( -21.15833593587365513, -24.48076211353314591, 80.99999999999991473 ) ) ;
#34096=EDGE_CURVE ( 'NONE', #30700, #14767, #33262, .T. ) ;
#34097=VECTOR ( 'NONE', #33926, 1000.000000000000000 ) ;
#34105=ORIENTED_EDGE ( 'NONE', *, *, #19154, .T. ) ;
#34111=ORIENTED_EDGE ( 'NONE', *, *, #2267, .T. ) ;
#34116=DIRECTION ( 'NONE',  ( 1.000000000000000000, 1.734723475976807094E-16, 0.000000000000000000 ) ) ;
#34130=CARTESIAN_POINT ( 'NONE',  ( -21.15833593587365513, -23.26666049839539951, 81.70096189432331357 ) ) ;
#34131=CARTESIAN_POINT ( 'NONE',  ( -34.49999999999998579, -30.19486372867100954, 85.70096189432321410 ) ) ;
#34142=PLANE ( 'NONE',  #10089 ) ;
#34143=CARTESIAN_POINT ( 'NONE',  ( -42.49999999999999289, -30.19486372867100954, 85.70096189432321410 ) ) ;
#34171=VECTOR ( 'NONE', #8623, 1000.000000000000000 ) ;
#34173=EDGE_CURVE ( 'NONE', #532, #27859, #27857, .T. ) ;
#34184=EDGE_CURVE ( 'NONE', #19677, #31595, #17204, .T. ) ;
#34194=VECTOR ( 'NONE', #26217, 1000.000000000000000 ) ;
#34199=VECTOR ( 'NONE', #168, 1000.000000000000000 ) ;
#34206=ORIENTED_EDGE ( 'NONE', *, *, #17614, .F. ) ;
#34234=VERTEX_POINT ( 'NONE', #20789 ) ;
#34248=PRODUCT ( 'Toothed Ratchet Brake Disc', 'Toothed Ratchet Brake Disc', '', ( #28578 ) ) ;
#34267=EDGE_LOOP ( 'NONE', ( #31968, #8962, #27075, #9637 ) ) ;
#34282=VERTEX_POINT ( 'NONE', #14867 ) ;
#34289=ORIENTED_EDGE ( 'NONE', *, *, #30631, .T. ) ;
#34295=EDGE_CURVE ( 'NONE', #34234, #26460, #34325, .T. ) ;
#34313=CARTESIAN_POINT ( 'NONE',  ( -42.49999999999999289, -41.45319397786874305, 92.20096189432315725 ) ) ;
#34323=EDGE_LOOP ( 'NONE', ( #5200, #713, #18872, #12929 ) ) ;
#34324=VERTEX_POINT ( 'NONE', #18460 ) ;
#34325=LINE ( 'NONE', #31440, #9034 ) ;
#34327=CARTESIAN_POINT ( 'NONE',  ( -42.49999999999999289, -22.68172400785658382, 87.71410161513770731 ) ) ;
#34331=EDGE_CURVE ( 'NONE', #2158, #19176, #34943, .T. ) ;
#34359=AXIS2_PLACEMENT_3D ( 'NONE', #34094, #22559, #30686 ) ;
#34375=CARTESIAN_POINT ( 'NONE',  ( -34.49999999999998579, -31.68172400785665488, 97.87435565298206086 ) ) ;
#34393=DIRECTION ( 'NONE',  ( 0.000000000000000000, 0.4999999999999898415, 0.8660254037844444808 ) ) ;
#34418=VECTOR ( 'NONE', #7983, 1000.000000000000000 ) ;
#34419=CARTESIAN_POINT ( 'NONE',  ( -34.49999999999998579, -38.85511776651532756, 79.29903810567645905 ) ) ;
#34428=EDGE_CURVE ( 'NONE', #35591, #25299, #24408, .T. ) ;
#34455=DIRECTION ( 'NONE',  ( 0.000000000000000000, 1.067522139062650474E-15, 1.000000000000000000 ) ) ;
#34475=ORIENTED_EDGE ( 'NONE', *, *, #6771, .F. ) ;
#34489=PRODUCT_DEFINITION_FORMATION_WITH_SPECIFIED_SOURCE ( 'ANY', '', #34248, .NOT_KNOWN. ) ;
#34503=ORIENTED_EDGE ( 'NONE', *, *, #34295, .T. ) ;
#34508=ORIENTED_EDGE ( 'NONE', *, *, #21274, .T. ) ;
#34522=DIRECTION ( 'NONE',  ( -1.000000000000000000, -1.734723475976807094E-16, -0.000000000000000000 ) ) ;
#34526=MANIFOLD_SOLID_BREP ( 'Cavity1', #5493 ) ;
#34548=ORIENTED_EDGE ( 'NONE', *, *, #27556, .F. ) ;
#34556=ORIENTED_EDGE ( 'NONE', *, *, #12991, .F. ) ;
#34590=CARTESIAN_POINT ( 'NONE',  ( -34.49999999999998579, -13.17619866229203396, 90.66066734786082293 ) ) ;
#34609=LINE ( 'NONE', #1292, #7491 ) ;
#34654=DIRECTION ( 'NONE',  ( 0.000000000000000000, 1.000000000000000000, 0.000000000000000000 ) ) ;
#34656=CIRCLE ( 'NONE', #19112, 14.00000000000000000 ) ;
#34675=CARTESIAN_POINT ( 'NONE',  ( -21.15833593587365513, -11.98076211353319742, 83.49999999999992895 ) ) ;
#34719=CARTESIAN_POINT ( 'NONE',  ( -34.50000000000001421, -41.45319397786874305, 92.20096189432315725 ) ) ;
#34723=CARTESIAN_POINT ( 'NONE',  ( -34.49999999999998579, -25.98076211353320986, 84.99999999999994316 ) ) ;
#34794=ADVANCED_FACE ( 'NONE', ( #29776 ), #24022, .F. ) ;
#34802=FACE_OUTER_BOUND ( 'NONE', #15802, .T. ) ;
#34805=FACE_OUTER_BOUND ( 'NONE', #14608, .T. ) ;
#34806=DIRECTION ( 'NONE',  ( -1.000000000000000000, 0.000000000000000000, 0.000000000000000000 ) ) ;
#34810=EDGE_LOOP ( 'NONE', ( #5606, #13558, #7325, #884 ) ) ;
#34826=VECTOR ( 'NONE', #18632, 1000.000000000000000 ) ;
#34831=EDGE_CURVE ( 'NONE', #26771, #20546, #21642, .T. ) ;
#34854=ORIENTED_EDGE ( 'NONE', *, *, #32457, .F. ) ;
#34863=CARTESIAN_POINT ( 'NONE',  ( -34.49999999999998579, -12.06135120645816272, 83.49999999999992895 ) ) ;
#34870=VERTEX_POINT ( 'NONE', #21826 ) ;
#34872=ORIENTED_EDGE ( 'NONE', *, *, #26507, .T. ) ;
#34897=DIRECTION ( 'NONE',  ( 0.000000000000000000, -0.8660254037844350439, -0.5000000000000061062 ) ) ;
#34943=CIRCLE ( 'NONE', #11917, 14.00000000000000000 ) ;
#34960=VECTOR ( 'NONE', #13767, 1000.000000000000000 ) ;
#34969=ADVANCED_FACE ( 'NONE', ( #11391 ), #5459, .F. ) ;
#34971=EDGE_LOOP ( 'NONE', ( #3894, #336, #35501, #22445, #35572, #32777, #33392, #10464, #31420, #17640, #11173, #11119, #33001, #32825, #12550, #30698, #20977, #22119, #18564, #9262, #25385, #1160, #6374, #32435, #34556, #25176, #9967, #22298, #29779, #16462, #1039, #10806, #34854, #14219, #34289, #19993, #22311, #31182, #5814, #17247, #16905, #31653, #11334, #22058, #6448, #29024, #27485, #24025 ) ) ;
#34982=ORIENTED_EDGE ( 'NONE', *, *, #2302, .T. ) ;
#34999=EDGE_CURVE ( 'NONE', #11172, #33126, #30817, .T. ) ;
#35018=DIRECTION ( 'NONE',  ( 0.000000000000000000, 0.9672551082808337197, -0.2538061376417689030 ) ) ;
#35019=VERTEX_POINT ( 'NONE', #30647 ) ;
#35049=DIRECTION ( 'NONE',  ( 0.000000000000000000, 1.000000000000000000, 0.000000000000000000 ) ) ;
#35055=DIRECTION ( 'NONE',  ( 1.226634733346697831E-16, -0.7071067811865557884, 0.7071067811865392461 ) ) ;
#35056=LINE ( 'NONE', #4631, #31211 ) ;
#35064=LINE ( 'NONE', #10386, #13747 ) ;
#35112=DIRECTION ( 'NONE',  ( -1.000000000000000000, 0.000000000000000000, 0.000000000000000000 ) ) ;
#35167=EDGE_LOOP ( 'NONE', ( #15926, #9988, #9776, #16401 ) ) ;
#35190=ORIENTED_EDGE ( 'NONE', *, *, #14757, .F. ) ;
#35201=CARTESIAN_POINT ( 'NONE',  ( -42.49999999999999289, -28.31857036507959791, 80.03062855292519373 ) ) ;
#35215=FACE_BOUND ( 'NONE', #24863, .T. ) ;
#35258=ORIENTED_EDGE ( 'NONE', *, *, #20032, .F. ) ;
#35274=DIRECTION ( 'NONE',  ( 0.000000000000000000, 2.423959199780483078E-15, -1.000000000000000000 ) ) ;
#35279=ORIENTED_EDGE ( 'NONE', *, *, #16794, .T. ) ;
#35284=DIRECTION ( 'NONE',  ( 0.000000000000000000, 1.000000000000000000, 0.000000000000000000 ) ) ;
#35396=DIRECTION ( 'NONE',  ( -1.000000000000000000, 1.502314598737152375E-16, 8.673617379884158732E-17 ) ) ;
#35405=CARTESIAN_POINT ( 'NONE',  ( -42.49999999999999289, -17.72201855431906736, 96.30456345124113682 ) ) ;
#35418=DIRECTION ( 'NONE',  ( -1.000000000000000000, 0.000000000000000000, 0.000000000000000000 ) ) ;
#35467=CARTESIAN_POINT ( 'NONE',  ( -42.49999999999999289, -25.98076211353322051, 84.99999999999992895 ) ) ;
#35483=ORIENTED_EDGE ( 'NONE', *, *, #19334, .T. ) ;
#35490=CARTESIAN_POINT ( 'NONE',  ( -34.49999999999998579, -25.98076211353322051, 84.99999999999992895 ) ) ;
#35495=EDGE_CURVE ( 'NONE', #10255, #18652, #22438, .T. ) ;
#35501=ORIENTED_EDGE ( 'NONE', *, *, #7670, .T. ) ;
#35527=LINE ( 'NONE', #14061, #23364 ) ;
#35551=CIRCLE ( 'NONE', #29695, 14.00000000000000000 ) ;
#35559=LINE ( 'NONE', #24565, #27448 ) ;
#35564=FACE_OUTER_BOUND ( 'NONE', #4902, .T. ) ;
#35572=ORIENTED_EDGE ( 'NONE', *, *, #20121, .F. ) ;
#35591=VERTEX_POINT ( 'NONE', #20794 ) ;
ENDSEC;
END-ISO-10303-21;
